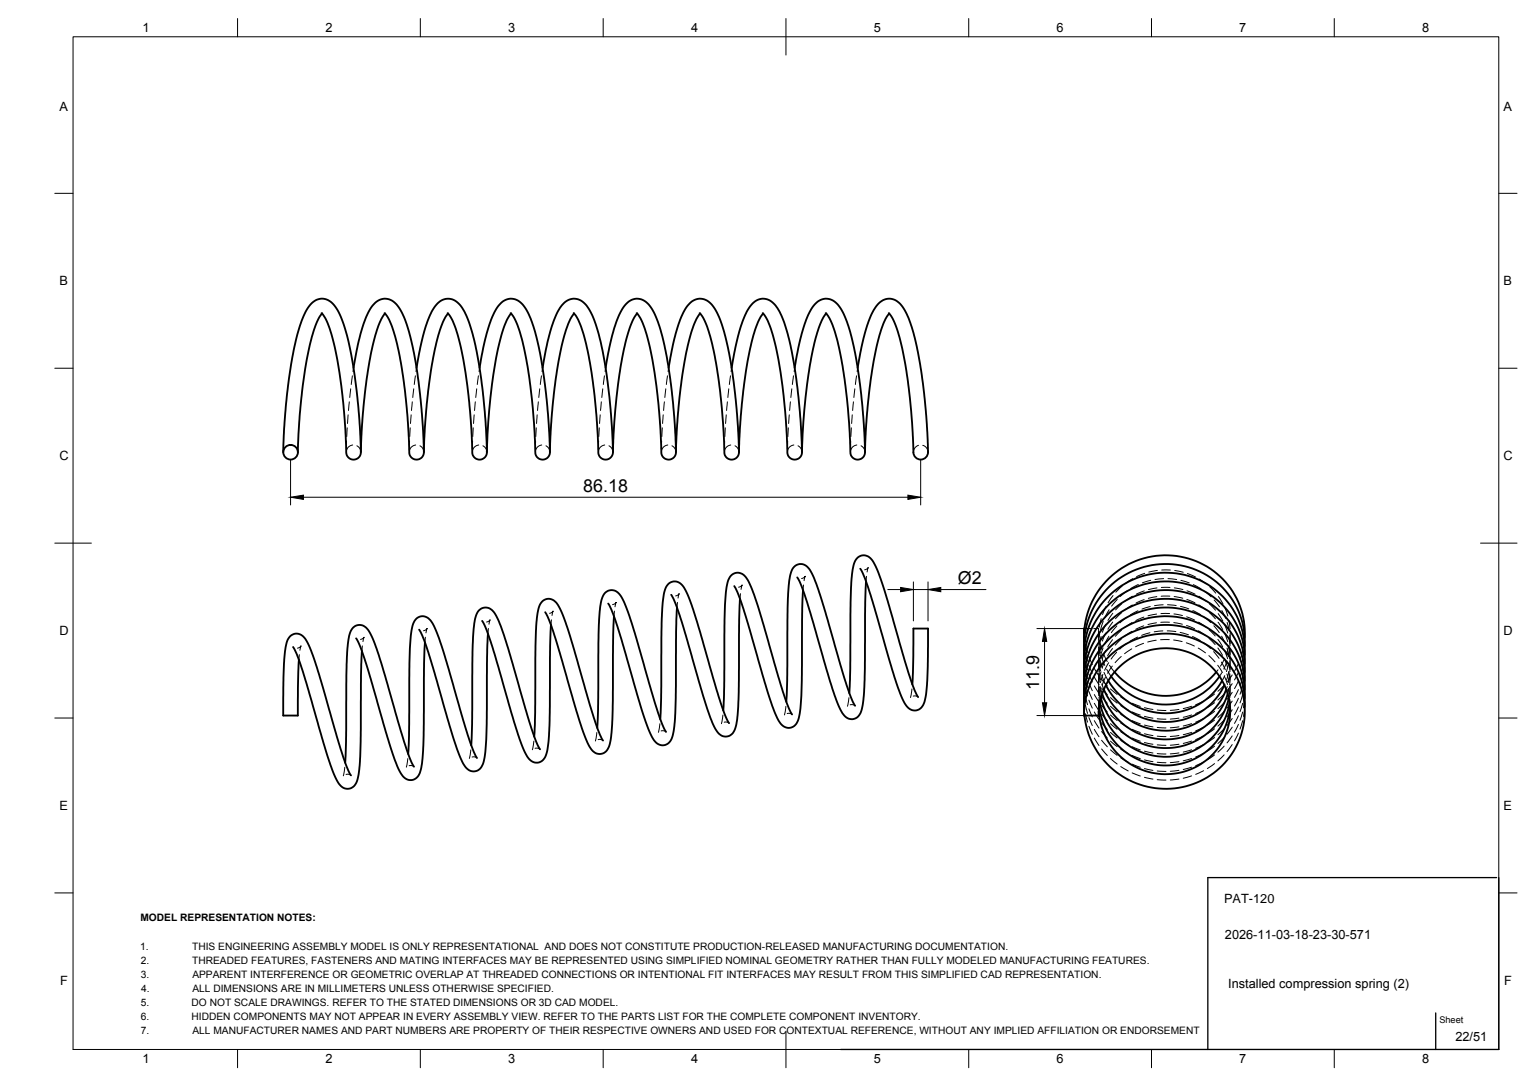
ISO-10303-21;
HEADER;
/* Generated by software containing ST-Developer
 * from STEP Tools, Inc. (www.steptools.com) 
 */

FILE_DESCRIPTION(
/* description */ ('Vibration shaker table dummy'),
/* implementation_level */ '2;1');

FILE_NAME(
/* name */ 'Installed compression spring (2).step',
/* time_stamp */ '2026-10-27T10:55:14-07:00',
/* author */ (''),
/* organization */ (''),
/* preprocessor_version */ 'ST-DEVELOPER v20.2',
/* originating_system */ 'Autodesk Translation Framework v15.17.0.0',
/* authorisation */ '');

FILE_SCHEMA (('AUTOMOTIVE_DESIGN { 1 0 10303 214 3 1 1 }'));
ENDSEC;

DATA;
#10=MECHANICAL_DESIGN_GEOMETRIC_PRESENTATION_REPRESENTATION('',(#703),#22394);
#588=B_SPLINE_CURVE_WITH_KNOTS('',3,(#19137,#19138,#19139,#19140,#19141,
#19142,#19143,#19144,#19145,#19146,#19147,#19148,#19149,#19150,#19151,#19152,
#19153,#19154,#19155,#19156,#19157,#19158,#19159,#19160,#19161,#19162,#19163,
#19164,#19165,#19166,#19167,#19168,#19169,#19170,#19171,#19172,#19173,#19174,
#19175,#19176,#19177,#19178,#19179,#19180,#19181,#19182,#19183,#19184,#19185,
#19186,#19187,#19188,#19189,#19190,#19191,#19192,#19193,#19194,#19195,#19196,
#19197,#19198,#19199,#19200,#19201,#19202,#19203,#19204,#19205,#19206,#19207,
#19208,#19209,#19210,#19211,#19212,#19213,#19214,#19215,#19216,#19217,#19218,
#19219,#19220,#19221,#19222,#19223,#19224,#19225,#19226,#19227,#19228,#19229,
#19230,#19231,#19232,#19233,#19234,#19235,#19236,#19237,#19238,#19239,#19240,
#19241,#19242,#19243,#19244,#19245,#19246,#19247,#19248,#19249,#19250,#19251,
#19252,#19253,#19254,#19255,#19256,#19257,#19258,#19259,#19260,#19261,#19262,
#19263,#19264,#19265,#19266,#19267,#19268,#19269,#19270,#19271,#19272,#19273,
#19274),.UNSPECIFIED.,.F.,.F.,(4,1,1,1,1,1,1,1,1,1,1,1,1,1,1,1,1,1,1,1,
1,1,1,1,1,1,1,1,1,1,1,1,1,1,1,1,1,1,1,1,1,1,1,1,1,1,1,1,1,1,1,1,1,1,1,1,
1,1,1,1,1,1,1,1,1,1,1,1,1,1,1,1,1,1,1,1,1,1,1,1,1,1,1,1,1,1,1,1,1,1,1,1,
1,1,1,1,1,1,1,1,1,1,1,1,1,1,1,1,1,1,1,1,1,1,1,1,1,1,1,1,1,1,1,1,1,1,1,1,
1,1,1,1,1,1,1,4),(0.,0.00892857142857143,0.0178571428571429,0.0267857142857143,
0.0357142857142857,0.0446428571428571,0.0535714285714286,0.0625,0.0714285714285714,
0.0803571428571428,0.0892857142857143,0.0982142857142857,0.107142857142857,
0.116071428571429,0.125,0.133928571428571,0.142857142857143,0.150793650793651,
0.154761904761905,0.156746031746032,0.158730158730159,0.166666666666667,
0.174603174603175,0.182539682539683,0.19047619047619,0.196428571428571,
0.202380952380952,0.208333333333333,0.214285714285714,0.222222222222222,
0.23015873015873,0.238095238095238,0.241071428571429,0.244047619047619,
0.25,0.255952380952381,0.261904761904762,0.267857142857143,0.273809523809524,
0.279761904761905,0.285714285714286,0.297619047619048,0.30952380952381,
0.321428571428571,0.327380952380952,0.333333333333333,0.341269841269841,
0.349206349206349,0.357142857142857,0.361111111111111,0.363095238095238,
0.365079365079365,0.373015873015873,0.380952380952381,0.386904761904762,
0.392857142857143,0.398809523809524,0.404761904761905,0.410714285714286,
0.416666666666667,0.422619047619048,0.428571428571429,0.4375,0.446428571428571,
0.455357142857143,0.459821428571429,0.464285714285714,0.470238095238095,
0.476190476190476,0.482142857142857,0.491071428571429,0.5,0.508928571428571,
0.517857142857143,0.526785714285714,0.535714285714286,0.544642857142857,
0.553571428571429,0.5625,0.571428571428571,0.580357142857143,0.589285714285714,
0.598214285714286,0.607142857142857,0.616071428571429,0.625,0.633928571428571,
0.642857142857143,0.650793650793651,0.658730158730159,0.666666666666667,
0.672619047619048,0.678571428571428,0.684523809523809,0.69047619047619,
0.696428571428571,0.702380952380952,0.708333333333333,0.714285714285714,
0.720238095238095,0.726190476190476,0.732142857142857,0.738095238095238,
0.744047619047619,0.75,0.755952380952381,0.761904761904762,0.76984126984127,
0.777777777777778,0.785714285714286,0.787946428571428,0.790178571428571,
0.794642857142857,0.803571428571428,0.8125,0.821428571428571,0.830357142857143,
0.839285714285714,0.848214285714286,0.857142857142857,0.866071428571429,
0.875,0.883928571428571,0.892857142857143,0.901785714285714,0.910714285714286,
0.919642857142857,0.928571428571429,0.9375,0.946428571428571,0.955357142857143,
0.964285714285714,0.973214285714286,0.982142857142857,0.991071428571429,
1.),.UNSPECIFIED.);
#592=B_SPLINE_SURFACE_WITH_KNOTS('',3,3,((#17754,#17755,#17756,#17757,#17758,
#17759,#17760,#17761,#17762,#17763,#17764,#17765,#17766,#17767,#17768,#17769,
#17770,#17771,#17772,#17773,#17774,#17775,#17776,#17777,#17778,#17779,#17780,
#17781,#17782,#17783,#17784,#17785,#17786,#17787,#17788,#17789,#17790,#17791,
#17792,#17793,#17794,#17795,#17796,#17797,#17798,#17799,#17800,#17801,#17802,
#17803,#17804,#17805,#17806,#17807,#17808,#17809,#17810,#17811,#17812,#17813,
#17814,#17815,#17816,#17817,#17818,#17819,#17820,#17821,#17822,#17823,#17824,
#17825,#17826,#17827,#17828,#17829,#17830,#17831,#17832,#17833,#17834,#17835,
#17836,#17837,#17838,#17839,#17840,#17841,#17842,#17843,#17844,#17845,#17846,
#17847,#17848,#17849,#17850,#17851,#17852,#17853,#17854,#17855,#17856,#17857,
#17858,#17859,#17860,#17861,#17862,#17863,#17864,#17865,#17866,#17867,#17868,
#17869,#17870,#17871,#17872,#17873,#17874,#17875,#17876,#17877,#17878,#17879,
#17880,#17881,#17882,#17883,#17884,#17885,#17886,#17887,#17888,#17889,#17890,
#17891),(#17892,#17893,#17894,#17895,#17896,#17897,#17898,#17899,#17900,
#17901,#17902,#17903,#17904,#17905,#17906,#17907,#17908,#17909,#17910,#17911,
#17912,#17913,#17914,#17915,#17916,#17917,#17918,#17919,#17920,#17921,#17922,
#17923,#17924,#17925,#17926,#17927,#17928,#17929,#17930,#17931,#17932,#17933,
#17934,#17935,#17936,#17937,#17938,#17939,#17940,#17941,#17942,#17943,#17944,
#17945,#17946,#17947,#17948,#17949,#17950,#17951,#17952,#17953,#17954,#17955,
#17956,#17957,#17958,#17959,#17960,#17961,#17962,#17963,#17964,#17965,#17966,
#17967,#17968,#17969,#17970,#17971,#17972,#17973,#17974,#17975,#17976,#17977,
#17978,#17979,#17980,#17981,#17982,#17983,#17984,#17985,#17986,#17987,#17988,
#17989,#17990,#17991,#17992,#17993,#17994,#17995,#17996,#17997,#17998,#17999,
#18000,#18001,#18002,#18003,#18004,#18005,#18006,#18007,#18008,#18009,#18010,
#18011,#18012,#18013,#18014,#18015,#18016,#18017,#18018,#18019,#18020,#18021,
#18022,#18023,#18024,#18025,#18026,#18027,#18028,#18029),(#18030,#18031,
#18032,#18033,#18034,#18035,#18036,#18037,#18038,#18039,#18040,#18041,#18042,
#18043,#18044,#18045,#18046,#18047,#18048,#18049,#18050,#18051,#18052,#18053,
#18054,#18055,#18056,#18057,#18058,#18059,#18060,#18061,#18062,#18063,#18064,
#18065,#18066,#18067,#18068,#18069,#18070,#18071,#18072,#18073,#18074,#18075,
#18076,#18077,#18078,#18079,#18080,#18081,#18082,#18083,#18084,#18085,#18086,
#18087,#18088,#18089,#18090,#18091,#18092,#18093,#18094,#18095,#18096,#18097,
#18098,#18099,#18100,#18101,#18102,#18103,#18104,#18105,#18106,#18107,#18108,
#18109,#18110,#18111,#18112,#18113,#18114,#18115,#18116,#18117,#18118,#18119,
#18120,#18121,#18122,#18123,#18124,#18125,#18126,#18127,#18128,#18129,#18130,
#18131,#18132,#18133,#18134,#18135,#18136,#18137,#18138,#18139,#18140,#18141,
#18142,#18143,#18144,#18145,#18146,#18147,#18148,#18149,#18150,#18151,#18152,
#18153,#18154,#18155,#18156,#18157,#18158,#18159,#18160,#18161,#18162,#18163,
#18164,#18165,#18166,#18167),(#18168,#18169,#18170,#18171,#18172,#18173,
#18174,#18175,#18176,#18177,#18178,#18179,#18180,#18181,#18182,#18183,#18184,
#18185,#18186,#18187,#18188,#18189,#18190,#18191,#18192,#18193,#18194,#18195,
#18196,#18197,#18198,#18199,#18200,#18201,#18202,#18203,#18204,#18205,#18206,
#18207,#18208,#18209,#18210,#18211,#18212,#18213,#18214,#18215,#18216,#18217,
#18218,#18219,#18220,#18221,#18222,#18223,#18224,#18225,#18226,#18227,#18228,
#18229,#18230,#18231,#18232,#18233,#18234,#18235,#18236,#18237,#18238,#18239,
#18240,#18241,#18242,#18243,#18244,#18245,#18246,#18247,#18248,#18249,#18250,
#18251,#18252,#18253,#18254,#18255,#18256,#18257,#18258,#18259,#18260,#18261,
#18262,#18263,#18264,#18265,#18266,#18267,#18268,#18269,#18270,#18271,#18272,
#18273,#18274,#18275,#18276,#18277,#18278,#18279,#18280,#18281,#18282,#18283,
#18284,#18285,#18286,#18287,#18288,#18289,#18290,#18291,#18292,#18293,#18294,
#18295,#18296,#18297,#18298,#18299,#18300,#18301,#18302,#18303,#18304,#18305),
(#18306,#18307,#18308,#18309,#18310,#18311,#18312,#18313,#18314,#18315,
#18316,#18317,#18318,#18319,#18320,#18321,#18322,#18323,#18324,#18325,#18326,
#18327,#18328,#18329,#18330,#18331,#18332,#18333,#18334,#18335,#18336,#18337,
#18338,#18339,#18340,#18341,#18342,#18343,#18344,#18345,#18346,#18347,#18348,
#18349,#18350,#18351,#18352,#18353,#18354,#18355,#18356,#18357,#18358,#18359,
#18360,#18361,#18362,#18363,#18364,#18365,#18366,#18367,#18368,#18369,#18370,
#18371,#18372,#18373,#18374,#18375,#18376,#18377,#18378,#18379,#18380,#18381,
#18382,#18383,#18384,#18385,#18386,#18387,#18388,#18389,#18390,#18391,#18392,
#18393,#18394,#18395,#18396,#18397,#18398,#18399,#18400,#18401,#18402,#18403,
#18404,#18405,#18406,#18407,#18408,#18409,#18410,#18411,#18412,#18413,#18414,
#18415,#18416,#18417,#18418,#18419,#18420,#18421,#18422,#18423,#18424,#18425,
#18426,#18427,#18428,#18429,#18430,#18431,#18432,#18433,#18434,#18435,#18436,
#18437,#18438,#18439,#18440,#18441,#18442,#18443),(#18444,#18445,#18446,
#18447,#18448,#18449,#18450,#18451,#18452,#18453,#18454,#18455,#18456,#18457,
#18458,#18459,#18460,#18461,#18462,#18463,#18464,#18465,#18466,#18467,#18468,
#18469,#18470,#18471,#18472,#18473,#18474,#18475,#18476,#18477,#18478,#18479,
#18480,#18481,#18482,#18483,#18484,#18485,#18486,#18487,#18488,#18489,#18490,
#18491,#18492,#18493,#18494,#18495,#18496,#18497,#18498,#18499,#18500,#18501,
#18502,#18503,#18504,#18505,#18506,#18507,#18508,#18509,#18510,#18511,#18512,
#18513,#18514,#18515,#18516,#18517,#18518,#18519,#18520,#18521,#18522,#18523,
#18524,#18525,#18526,#18527,#18528,#18529,#18530,#18531,#18532,#18533,#18534,
#18535,#18536,#18537,#18538,#18539,#18540,#18541,#18542,#18543,#18544,#18545,
#18546,#18547,#18548,#18549,#18550,#18551,#18552,#18553,#18554,#18555,#18556,
#18557,#18558,#18559,#18560,#18561,#18562,#18563,#18564,#18565,#18566,#18567,
#18568,#18569,#18570,#18571,#18572,#18573,#18574,#18575,#18576,#18577,#18578,
#18579,#18580,#18581),(#18582,#18583,#18584,#18585,#18586,#18587,#18588,
#18589,#18590,#18591,#18592,#18593,#18594,#18595,#18596,#18597,#18598,#18599,
#18600,#18601,#18602,#18603,#18604,#18605,#18606,#18607,#18608,#18609,#18610,
#18611,#18612,#18613,#18614,#18615,#18616,#18617,#18618,#18619,#18620,#18621,
#18622,#18623,#18624,#18625,#18626,#18627,#18628,#18629,#18630,#18631,#18632,
#18633,#18634,#18635,#18636,#18637,#18638,#18639,#18640,#18641,#18642,#18643,
#18644,#18645,#18646,#18647,#18648,#18649,#18650,#18651,#18652,#18653,#18654,
#18655,#18656,#18657,#18658,#18659,#18660,#18661,#18662,#18663,#18664,#18665,
#18666,#18667,#18668,#18669,#18670,#18671,#18672,#18673,#18674,#18675,#18676,
#18677,#18678,#18679,#18680,#18681,#18682,#18683,#18684,#18685,#18686,#18687,
#18688,#18689,#18690,#18691,#18692,#18693,#18694,#18695,#18696,#18697,#18698,
#18699,#18700,#18701,#18702,#18703,#18704,#18705,#18706,#18707,#18708,#18709,
#18710,#18711,#18712,#18713,#18714,#18715,#18716,#18717,#18718,#18719),
(#18720,#18721,#18722,#18723,#18724,#18725,#18726,#18727,#18728,#18729,
#18730,#18731,#18732,#18733,#18734,#18735,#18736,#18737,#18738,#18739,#18740,
#18741,#18742,#18743,#18744,#18745,#18746,#18747,#18748,#18749,#18750,#18751,
#18752,#18753,#18754,#18755,#18756,#18757,#18758,#18759,#18760,#18761,#18762,
#18763,#18764,#18765,#18766,#18767,#18768,#18769,#18770,#18771,#18772,#18773,
#18774,#18775,#18776,#18777,#18778,#18779,#18780,#18781,#18782,#18783,#18784,
#18785,#18786,#18787,#18788,#18789,#18790,#18791,#18792,#18793,#18794,#18795,
#18796,#18797,#18798,#18799,#18800,#18801,#18802,#18803,#18804,#18805,#18806,
#18807,#18808,#18809,#18810,#18811,#18812,#18813,#18814,#18815,#18816,#18817,
#18818,#18819,#18820,#18821,#18822,#18823,#18824,#18825,#18826,#18827,#18828,
#18829,#18830,#18831,#18832,#18833,#18834,#18835,#18836,#18837,#18838,#18839,
#18840,#18841,#18842,#18843,#18844,#18845,#18846,#18847,#18848,#18849,#18850,
#18851,#18852,#18853,#18854,#18855,#18856,#18857),(#18858,#18859,#18860,
#18861,#18862,#18863,#18864,#18865,#18866,#18867,#18868,#18869,#18870,#18871,
#18872,#18873,#18874,#18875,#18876,#18877,#18878,#18879,#18880,#18881,#18882,
#18883,#18884,#18885,#18886,#18887,#18888,#18889,#18890,#18891,#18892,#18893,
#18894,#18895,#18896,#18897,#18898,#18899,#18900,#18901,#18902,#18903,#18904,
#18905,#18906,#18907,#18908,#18909,#18910,#18911,#18912,#18913,#18914,#18915,
#18916,#18917,#18918,#18919,#18920,#18921,#18922,#18923,#18924,#18925,#18926,
#18927,#18928,#18929,#18930,#18931,#18932,#18933,#18934,#18935,#18936,#18937,
#18938,#18939,#18940,#18941,#18942,#18943,#18944,#18945,#18946,#18947,#18948,
#18949,#18950,#18951,#18952,#18953,#18954,#18955,#18956,#18957,#18958,#18959,
#18960,#18961,#18962,#18963,#18964,#18965,#18966,#18967,#18968,#18969,#18970,
#18971,#18972,#18973,#18974,#18975,#18976,#18977,#18978,#18979,#18980,#18981,
#18982,#18983,#18984,#18985,#18986,#18987,#18988,#18989,#18990,#18991,#18992,
#18993,#18994,#18995),(#18996,#18997,#18998,#18999,#19000,#19001,#19002,
#19003,#19004,#19005,#19006,#19007,#19008,#19009,#19010,#19011,#19012,#19013,
#19014,#19015,#19016,#19017,#19018,#19019,#19020,#19021,#19022,#19023,#19024,
#19025,#19026,#19027,#19028,#19029,#19030,#19031,#19032,#19033,#19034,#19035,
#19036,#19037,#19038,#19039,#19040,#19041,#19042,#19043,#19044,#19045,#19046,
#19047,#19048,#19049,#19050,#19051,#19052,#19053,#19054,#19055,#19056,#19057,
#19058,#19059,#19060,#19061,#19062,#19063,#19064,#19065,#19066,#19067,#19068,
#19069,#19070,#19071,#19072,#19073,#19074,#19075,#19076,#19077,#19078,#19079,
#19080,#19081,#19082,#19083,#19084,#19085,#19086,#19087,#19088,#19089,#19090,
#19091,#19092,#19093,#19094,#19095,#19096,#19097,#19098,#19099,#19100,#19101,
#19102,#19103,#19104,#19105,#19106,#19107,#19108,#19109,#19110,#19111,#19112,
#19113,#19114,#19115,#19116,#19117,#19118,#19119,#19120,#19121,#19122,#19123,
#19124,#19125,#19126,#19127,#19128,#19129,#19130,#19131,#19132,#19133)),
 .UNSPECIFIED.,.T.,.F.,.F.,(4,1,1,1,1,1,1,4),(4,1,1,1,1,1,1,1,1,1,1,1,1,
1,1,1,1,1,1,1,1,1,1,1,1,1,1,1,1,1,1,1,1,1,1,1,1,1,1,1,1,1,1,1,1,1,1,1,1,
1,1,1,1,1,1,1,1,1,1,1,1,1,1,1,1,1,1,1,1,1,1,1,1,1,1,1,1,1,1,1,1,1,1,1,1,
1,1,1,1,1,1,1,1,1,1,1,1,1,1,1,1,1,1,1,1,1,1,1,1,1,1,1,1,1,1,1,1,1,1,1,1,
1,1,1,1,1,1,1,1,1,1,1,1,1,1,4),(-3.14159265358979,-2.24399475256414,-1.34639685153848,
-0.448798950512828,0.448798950512828,1.34639685153848,2.24399475256414,
3.14159265358979),(0.,0.00892857142857143,0.0178571428571429,0.0267857142857143,
0.0357142857142857,0.0446428571428571,0.0535714285714286,0.0625,0.0714285714285714,
0.0803571428571428,0.0892857142857143,0.0982142857142857,0.107142857142857,
0.116071428571429,0.125,0.133928571428571,0.142857142857143,0.150793650793651,
0.154761904761905,0.156746031746032,0.158730158730159,0.166666666666667,
0.174603174603175,0.182539682539683,0.19047619047619,0.196428571428571,
0.202380952380952,0.208333333333333,0.214285714285714,0.222222222222222,
0.23015873015873,0.238095238095238,0.241071428571429,0.244047619047619,
0.25,0.255952380952381,0.261904761904762,0.267857142857143,0.273809523809524,
0.279761904761905,0.285714285714286,0.297619047619048,0.30952380952381,
0.321428571428571,0.327380952380952,0.333333333333333,0.341269841269841,
0.349206349206349,0.357142857142857,0.361111111111111,0.363095238095238,
0.365079365079365,0.373015873015873,0.380952380952381,0.386904761904762,
0.392857142857143,0.398809523809524,0.404761904761905,0.410714285714286,
0.416666666666667,0.422619047619048,0.428571428571429,0.4375,0.446428571428571,
0.455357142857143,0.459821428571429,0.464285714285714,0.470238095238095,
0.476190476190476,0.482142857142857,0.491071428571429,0.5,0.508928571428571,
0.517857142857143,0.526785714285714,0.535714285714286,0.544642857142857,
0.553571428571429,0.5625,0.571428571428571,0.580357142857143,0.589285714285714,
0.598214285714286,0.607142857142857,0.616071428571429,0.625,0.633928571428571,
0.642857142857143,0.650793650793651,0.658730158730159,0.666666666666667,
0.672619047619048,0.678571428571428,0.684523809523809,0.69047619047619,
0.696428571428571,0.702380952380952,0.708333333333333,0.714285714285714,
0.720238095238095,0.726190476190476,0.732142857142857,0.738095238095238,
0.744047619047619,0.75,0.755952380952381,0.761904761904762,0.76984126984127,
0.777777777777778,0.785714285714286,0.787946428571428,0.790178571428571,
0.794642857142857,0.803571428571428,0.8125,0.821428571428571,0.830357142857143,
0.839285714285714,0.848214285714286,0.857142857142857,0.866071428571429,
0.875,0.883928571428571,0.892857142857143,0.901785714285714,0.910714285714286,
0.919642857142857,0.928571428571429,0.9375,0.946428571428571,0.955357142857143,
0.964285714285714,0.973214285714286,0.982142857142857,0.991071428571429,
1.),.UNSPECIFIED.);
#611=SHAPE_REPRESENTATION_RELATIONSHIP('SRR','None',#22657,#657);
#657=ADVANCED_BREP_SHAPE_REPRESENTATION('',(#749),#22363);
#703=STYLED_ITEM('',(#22961),#749);
#749=MANIFOLD_SOLID_BREP('Body1',#9221);
#1168=PLANE('',#10140);
#1169=PLANE('',#10141);
#1529=FACE_OUTER_BOUND('',#2157,.T.);
#1530=FACE_OUTER_BOUND('',#2158,.T.);
#1531=FACE_OUTER_BOUND('',#2159,.T.);
#2157=EDGE_LOOP('',(#7122,#7123,#7124,#7125));
#2158=EDGE_LOOP('',(#7126));
#2159=EDGE_LOOP('',(#7127));
#4032=CIRCLE('',#10138,0.1);
#4033=CIRCLE('',#10139,0.1);
#4659=VERTEX_POINT('',#19134);
#4660=VERTEX_POINT('',#19136);
#5554=EDGE_CURVE('',#4659,#4659,#4032,.T.);
#5555=EDGE_CURVE('',#4659,#4660,#588,.T.);
#5556=EDGE_CURVE('',#4660,#4660,#4033,.T.);
#7122=ORIENTED_EDGE('',*,*,#5554,.T.);
#7123=ORIENTED_EDGE('',*,*,#5555,.T.);
#7124=ORIENTED_EDGE('',*,*,#5556,.F.);
#7125=ORIENTED_EDGE('',*,*,#5555,.F.);
#7126=ORIENTED_EDGE('',*,*,#5556,.T.);
#7127=ORIENTED_EDGE('',*,*,#5554,.F.);
#8894=ADVANCED_FACE('',(#1529),#592,.T.);
#8895=ADVANCED_FACE('',(#1530),#1168,.T.);
#8896=ADVANCED_FACE('',(#1531),#1169,.F.);
#9221=CLOSED_SHELL('',(#8894,#8895,#8896));
#10137=AXIS2_PLACEMENT_3D('',#17753,#11968,#11969);
#10138=AXIS2_PLACEMENT_3D('',#19135,#11970,#11971);
#10139=AXIS2_PLACEMENT_3D('',#19275,#11972,#11973);
#10140=AXIS2_PLACEMENT_3D('',#19276,#11974,#11975);
#10141=AXIS2_PLACEMENT_3D('',#19277,#11976,#11977);
#11968=DIRECTION('axis',(0.,0.,1.));
#11969=DIRECTION('refdir',(1.,0.,0.));
#11970=DIRECTION('center_axis',(-0.000133356257939316,0.990604928518337,
0.136754735973894));
#11971=DIRECTION('ref_axis',(1.84100635426204E-5,-0.136754734734703,0.990604937494615));
#11972=DIRECTION('center_axis',(0.000133356514931307,0.990604928490669,
0.136754736174063));
#11973=DIRECTION('ref_axis',(-0.722226697922822,0.0946826992832939,-0.68514508190888));
#11974=DIRECTION('center_axis',(0.000133356514931307,0.990604928490669,
0.136754736174063));
#11975=DIRECTION('ref_axis',(-0.722226697922822,0.0946826992832939,-0.68514508190888));
#11976=DIRECTION('center_axis',(-0.000133356257939316,0.990604928518337,
0.136754735973894));
#11977=DIRECTION('ref_axis',(1.84100635426204E-5,-0.136754734734703,0.990604937494615));
#17753=CARTESIAN_POINT('',(0.,0.,0.));
#17754=CARTESIAN_POINT('Ctrl Pts',(6.99999815899365,-3.98632452652653,2.60093950625054));
#17755=CARTESIAN_POINT('Ctrl Pts',(6.99997288064459,-3.79855038269031,2.62686205390176));
#17756=CARTESIAN_POINT('Ctrl Pts',(6.89233514047511,-3.42414397295474,2.67881370715146));
#17757=CARTESIAN_POINT('Ctrl Pts',(6.45271448161715,-3.02998089899105,2.757384351524));
#17758=CARTESIAN_POINT('Ctrl Pts',(5.86671979479608,-2.93006055988124,2.83651312593273));
#17759=CARTESIAN_POINT('Ctrl Pts',(5.31329781017118,-3.15858496371257,2.91622300969429));
#17760=CARTESIAN_POINT('Ctrl Pts',(4.9638387202763,-3.65012742948249,2.99648818069946));
#17761=CARTESIAN_POINT('Ctrl Pts',(4.9293710419426,-4.25616717719541,3.07729927110974));
#17762=CARTESIAN_POINT('Ctrl Pts',(5.22419213535424,-4.79140012919127,3.15863486906283));
#17763=CARTESIAN_POINT('Ctrl Pts',(5.76222069265107,-5.08919945404236,3.24047453667969));
#17764=CARTESIAN_POINT('Ctrl Pts',(6.379677030618,-5.05504702300603,3.32279319426342));
#17765=CARTESIAN_POINT('Ctrl Pts',(6.88712884688249,-4.6955749219134,3.40556355651458));
#17766=CARTESIAN_POINT('Ctrl Pts',(7.12670085302573,-4.11831918936923,3.48875539197247));
#17767=CARTESIAN_POINT('Ctrl Pts',(7.02192637673817,-3.49920475943206,3.57233609217612));
#17768=CARTESIAN_POINT('Ctrl Pts',(6.60200480535371,-3.02877356919622,3.65627071403784));
#17769=CARTESIAN_POINT('Ctrl Pts',(5.99389696970595,-2.85326346917548,3.74052223770667));
#17770=CARTESIAN_POINT('Ctrl Pts',(5.38356210524816,-3.02876561374954,3.82505176545516));
#17771=CARTESIAN_POINT('Ctrl Pts',(4.97486808401256,-3.48597581907603,3.90667922332894));
#17772=CARTESIAN_POINT('Ctrl Pts',(4.87764331063032,-3.96854834063101,3.97275270796177));
#17773=CARTESIAN_POINT('Ctrl Pts',(4.93363491104256,-4.28466096216571,4.01685604464165));
#17774=CARTESIAN_POINT('Ctrl Pts',(4.99817931143911,-4.45530970670709,4.04207155735716));
#17775=CARTESIAN_POINT('Ctrl Pts',(5.12597275373369,-4.69744865131441,4.07990746653167));
#17776=CARTESIAN_POINT('Ctrl Pts',(5.42875069944469,-4.99309340796393,4.13670511444809));
#17777=CARTESIAN_POINT('Ctrl Pts',(5.97231920216535,-5.14605898976926,4.21249748606625));
#17778=CARTESIAN_POINT('Ctrl Pts',(6.52320508223107,-5.02044374257342,4.28832048254892));
#17779=CARTESIAN_POINT('Ctrl Pts',(6.91110467076896,-4.67743260856581,4.35782392841035));
#17780=CARTESIAN_POINT('Ctrl Pts',(7.09644745188598,-4.25185787791867,4.42098501720712));
#17781=CARTESIAN_POINT('Ctrl Pts',(7.11227598252982,-3.83457932502243,4.47779828333078));
#17782=CARTESIAN_POINT('Ctrl Pts',(6.97422198867159,-3.44096105119827,4.53456659991209));
#17783=CARTESIAN_POINT('Ctrl Pts',(6.67241777459347,-3.08955752755044,4.59757801617794));
#17784=CARTESIAN_POINT('Ctrl Pts',(6.20242890124212,-2.8776477149725,4.66678930738527));
#17785=CARTESIAN_POINT('Ctrl Pts',(5.64251878205079,-2.91980762281901,4.74213608937642));
#17786=CARTESIAN_POINT('Ctrl Pts',(5.2704159386044,-3.1605530148329,4.80163845364204));
#17787=CARTESIAN_POINT('Ctrl Pts',(5.0774166278585,-3.41255654376288,4.84539629257686));
#17788=CARTESIAN_POINT('Ctrl Pts',(4.95479769651029,-3.65506677262475,4.88286085266752));
#17789=CARTESIAN_POINT('Ctrl Pts',(4.89096164216428,-3.99267527518354,4.9296088561907));
#17790=CARTESIAN_POINT('Ctrl Pts',(4.9676452372308,-4.39667000889553,4.98556279567646));
#17791=CARTESIAN_POINT('Ctrl Pts',(5.18583996189851,-4.74396038265063,5.04136211338706));
#17792=CARTESIAN_POINT('Ctrl Pts',(5.51489715544512,-4.98648283834255,5.09699623582978));
#17793=CARTESIAN_POINT('Ctrl Pts',(5.90877797642046,-5.0921366099034,5.15245506500268));
#17794=CARTESIAN_POINT('Ctrl Pts',(6.31208382647452,-5.04618505638536,5.20772889790527));
#17795=CARTESIAN_POINT('Ctrl Pts',(6.79039563711824,-4.79482787477752,5.28116853494519));
#17796=CARTESIAN_POINT('Ctrl Pts',(7.14364250607538,-4.18339760328549,5.37246079320281));
#17797=CARTESIAN_POINT('Ctrl Pts',(6.95465392442801,-3.3615290602033,5.48113680479085));
#17798=CARTESIAN_POINT('Ctrl Pts',(6.37954281770185,-2.97211167108618,5.57092649504958));
#17799=CARTESIAN_POINT('Ctrl Pts',(5.85508217241069,-2.95446460563552,5.64227218334414));
#17800=CARTESIAN_POINT('Ctrl Pts',(5.44460306454923,-3.0974244576334,5.70145206942602));
#17801=CARTESIAN_POINT('Ctrl Pts',(5.09938139322235,-3.43453521092238,5.76619150122483));
#17802=CARTESIAN_POINT('Ctrl Pts',(4.94592320318296,-3.93442474869926,5.83636208316637));
#17803=CARTESIAN_POINT('Ctrl Pts',(5.03197265676116,-4.35840627465708,5.89445465107149));
#17804=CARTESIAN_POINT('Ctrl Pts',(5.19219264369348,-4.60564299044654,5.93491706685731));
#17805=CARTESIAN_POINT('Ctrl Pts',(5.30719577297855,-4.72651611720447,5.95798055540973));
#17806=CARTESIAN_POINT('Ctrl Pts',(5.50053046023923,-4.88495348501329,5.99251787759586));
#17807=CARTESIAN_POINT('Ctrl Pts',(5.85832951556707,-5.02507253962729,6.04410658286047));
#17808=CARTESIAN_POINT('Ctrl Pts',(6.32126493019694,-4.96668267597821,6.10673564915363));
#17809=CARTESIAN_POINT('Ctrl Pts',(6.67328517320073,-4.74489735077078,6.1633365491453));
#17810=CARTESIAN_POINT('Ctrl Pts',(6.89435900913716,-4.44516759248262,6.21402149084589));
#17811=CARTESIAN_POINT('Ctrl Pts',(6.99016055458223,-4.08705298460299,6.26445344730346));
#17812=CARTESIAN_POINT('Ctrl Pts',(6.94870527391535,-3.72056310115263,6.31463598339954));
#17813=CARTESIAN_POINT('Ctrl Pts',(6.77696548585144,-3.39623351183634,6.36457330966794));
#17814=CARTESIAN_POINT('Ctrl Pts',(6.50006848678236,-3.15797695360399,6.41427030439494));
#17815=CARTESIAN_POINT('Ctrl Pts',(6.15689079921747,-3.03828948600061,6.46373243937456));
#17816=CARTESIAN_POINT('Ctrl Pts',(5.73494713487383,-3.05387392617641,6.52117143017342));
#17817=CARTESIAN_POINT('Ctrl Pts',(5.30575107583077,-3.29070893773119,6.58644590514151));
#17818=CARTESIAN_POINT('Ctrl Pts',(5.04125313845857,-3.77122732190886,6.6594050878354));
#17819=CARTESIAN_POINT('Ctrl Pts',(5.06714113786846,-4.2240700226978,6.71983222627245));
#17820=CARTESIAN_POINT('Ctrl Pts',(5.22896371026909,-4.53583531846688,6.76796591127916));
#17821=CARTESIAN_POINT('Ctrl Pts',(5.42916113979845,-4.74785467675554,6.80796630808184));
#17822=CARTESIAN_POINT('Ctrl Pts',(5.714367370309,-4.89850759732021,6.85183024025803));
#17823=CARTESIAN_POINT('Ctrl Pts',(6.06253639457921,-4.93755475445945,6.89952195690528));
#17824=CARTESIAN_POINT('Ctrl Pts',(6.4565847787629,-4.83233977440753,6.95498839066731));
#17825=CARTESIAN_POINT('Ctrl Pts',(6.81022730237302,-4.51633849133825,7.01814871600544));
#17826=CARTESIAN_POINT('Ctrl Pts',(6.95706828830077,-4.00489886911992,7.08893287981098));
#17827=CARTESIAN_POINT('Ctrl Pts',(6.81021224891959,-3.49584469103884,7.15948666255227));
#17828=CARTESIAN_POINT('Ctrl Pts',(6.41592301667082,-3.14352189275395,7.22985222727915));
#17829=CARTESIAN_POINT('Ctrl Pts',(5.89582428767248,-3.0555832223308,7.30007283378182));
#17830=CARTESIAN_POINT('Ctrl Pts',(5.40914881608276,-3.25711226719962,7.37019262219717));
#17831=CARTESIAN_POINT('Ctrl Pts',(5.10471600640629,-3.68647088534127,7.4402563254545));
#17832=CARTESIAN_POINT('Ctrl Pts',(5.07493689936822,-4.21187381141773,7.51030900528994));
#17833=CARTESIAN_POINT('Ctrl Pts',(5.32972438815395,-4.67276168571651,7.58039577687912));
#17834=CARTESIAN_POINT('Ctrl Pts',(5.79102554371443,-4.92784792737786,7.65056157421906));
#17835=CARTESIAN_POINT('Ctrl Pts',(6.31826031255578,-4.89837953861158,7.72085085714204));
#17836=CARTESIAN_POINT('Ctrl Pts',(6.75020660471299,-4.59231290695902,7.79130734550421));
#17837=CARTESIAN_POINT('Ctrl Pts',(6.95334524231267,-4.10180979072915,7.86197377515194));
#17838=CARTESIAN_POINT('Ctrl Pts',(6.86452811856373,-3.57660445666216,7.93289164673106));
#17839=CARTESIAN_POINT('Ctrl Pts',(6.50822949801913,-3.17741851765368,8.00410096472273));
#17840=CARTESIAN_POINT('Ctrl Pts',(5.99202912111436,-3.02846879700038,8.07564001126929));
#17841=CARTESIAN_POINT('Ctrl Pts',(5.47262775862424,-3.1772786287127,8.14754510192845));
#17842=CARTESIAN_POINT('Ctrl Pts',(5.12396773984527,-3.56713104102442,8.21717245978697));
#17843=CARTESIAN_POINT('Ctrl Pts',(5.02465088008016,-4.0589090579052,8.28449962671212));
#17844=CARTESIAN_POINT('Ctrl Pts',(5.16664179671633,-4.52183049710153,8.34949563002517));
#17845=CARTESIAN_POINT('Ctrl Pts',(5.48622133819085,-4.83366725020512,8.40942447534479));
#17846=CARTESIAN_POINT('Ctrl Pts',(5.86625745021743,-4.9665851067969,8.4641954747342));
#17847=CARTESIAN_POINT('Ctrl Pts',(6.22997586892847,-4.95324406413884,8.5137197914407));
#17848=CARTESIAN_POINT('Ctrl Pts',(6.56523678307791,-4.80705258085916,8.56348049146453));
#17849=CARTESIAN_POINT('Ctrl Pts',(6.8252178463785,-4.54733568382595,8.61348288991823));
#17850=CARTESIAN_POINT('Ctrl Pts',(6.97306928054101,-4.20890471076454,8.6637316832973));
#17851=CARTESIAN_POINT('Ctrl Pts',(6.98712341108126,-3.83802816814003,8.7142309149468));
#17852=CARTESIAN_POINT('Ctrl Pts',(6.86409431800442,-3.4858887373625,8.76498396878373));
#17853=CARTESIAN_POINT('Ctrl Pts',(6.61968641501593,-3.20161333099039,8.81599356080702));
#17854=CARTESIAN_POINT('Ctrl Pts',(6.28663539552411,-3.02539046352671,8.8672617337013));
#17855=CARTESIAN_POINT('Ctrl Pts',(5.91032079687008,-2.98281618785264,8.9187898484193));
#17856=CARTESIAN_POINT('Ctrl Pts',(5.54261902100133,-3.08115683102349,8.97057858319571));
#17857=CARTESIAN_POINT('Ctrl Pts',(5.23470149593991,-3.30818973404657,9.02262792887906));
#17858=CARTESIAN_POINT('Ctrl Pts',(5.03002953653242,-3.63360637314209,9.07493719454492));
#17859=CARTESIAN_POINT('Ctrl Pts',(4.95795339049146,-4.01324887545392,9.12750499722226));
#17860=CARTESIAN_POINT('Ctrl Pts',(5.03008733681497,-4.39465616925505,9.18032929191999));
#17861=CARTESIAN_POINT('Ctrl Pts',(5.26037098227884,-4.76198737973904,9.23930488376548));
#17862=CARTESIAN_POINT('Ctrl Pts',(5.66815402132354,-5.02611715334513,9.30453505328307));
#17863=CARTESIAN_POINT('Ctrl Pts',(6.20031175950905,-5.06610553161693,9.37613052247429));
#17864=CARTESIAN_POINT('Ctrl Pts',(6.57211483447548,-4.89867154701958,9.43089482659667));
#17865=CARTESIAN_POINT('Ctrl Pts',(6.77268428325753,-4.71398594666241,9.46854124254023));
#17866=CARTESIAN_POINT('Ctrl Pts',(6.89732261541234,-4.56210906285714,9.4956893772699));
#17867=CARTESIAN_POINT('Ctrl Pts',(7.05743952416135,-4.25373892219051,9.54330952558428));
#17868=CARTESIAN_POINT('Ctrl Pts',(7.08681427060224,-3.7413976498585,9.61164803498953));
#17869=CARTESIAN_POINT('Ctrl Pts',(6.78743967682059,-3.19877575055479,9.69412425474241));
#17870=CARTESIAN_POINT('Ctrl Pts',(6.24245837315985,-2.89706443193603,9.77704206668623));
#17871=CARTESIAN_POINT('Ctrl Pts',(5.61746900273164,-2.93185417099466,9.86037047868398));
#17872=CARTESIAN_POINT('Ctrl Pts',(5.1042042416184,-3.29518411512121,9.94407604361117));
#17873=CARTESIAN_POINT('Ctrl Pts',(4.86233946758306,-3.8785536270643,10.0281231251224));
#17874=CARTESIAN_POINT('Ctrl Pts',(4.96816269898698,-4.50332086698013,10.1124740074888));
#17875=CARTESIAN_POINT('Ctrl Pts',(5.3915816199262,-4.97752738430232,10.1970892227568));
#17876=CARTESIAN_POINT('Ctrl Pts',(6.00397807691952,-5.15417755509278,10.281927720062));
#17877=CARTESIAN_POINT('Ctrl Pts',(6.61779621608409,-4.97752665860305,10.3669471357688));
#17878=CARTESIAN_POINT('Ctrl Pts',(7.04418758947222,-4.50057596349951,10.4521040140405));
#17879=CARTESIAN_POINT('Ctrl Pts',(7.15154318711507,-3.86917823804319,10.5373541207604));
#17880=CARTESIAN_POINT('Ctrl Pts',(6.9063217242137,-3.27712490715728,10.622652644332));
#17881=CARTESIAN_POINT('Ctrl Pts',(6.38365961018741,-2.90630232377856,10.70795449752));
#17882=CARTESIAN_POINT('Ctrl Pts',(5.74407957751689,-2.87046702674317,10.7932145497474));
#17883=CARTESIAN_POINT('Ctrl Pts',(5.18413779010185,-3.18009512220889,10.8783879953558));
#17884=CARTESIAN_POINT('Ctrl Pts',(4.87504525063398,-3.73939474085648,10.9634303821887));
#17885=CARTESIAN_POINT('Ctrl Pts',(4.9113280193628,-4.37593360867611,11.0482983399598));
#17886=CARTESIAN_POINT('Ctrl Pts',(5.27937248430205,-4.89450749674953,11.1329488708158));
#17887=CARTESIAN_POINT('Ctrl Pts',(5.86527624347711,-5.13679808752952,11.2173417295453));
#17888=CARTESIAN_POINT('Ctrl Pts',(6.48799534199112,-5.03087191620999,11.3014349903219));
#17889=CARTESIAN_POINT('Ctrl Pts',(6.95693136473707,-4.61090781293032,11.3851957485584));
#17890=CARTESIAN_POINT('Ctrl Pts',(7.07219562678886,-4.21035033769926,11.4407823887657));
#17891=CARTESIAN_POINT('Ctrl Pts',(7.07222266979228,-4.00946826992833,11.4685145081909));
#17892=CARTESIAN_POINT('Ctrl Pts',(6.97007822923057,-3.98632855437836,2.60093950625054));
#17893=CARTESIAN_POINT('Ctrl Pts',(6.97005368434428,-3.80400276250044,2.62610989942311));
#17894=CARTESIAN_POINT('Ctrl Pts',(6.8655981616237,-3.44058276592777,2.67653039560817));
#17895=CARTESIAN_POINT('Ctrl Pts',(6.43867935390673,-3.05771294402619,2.75283688635242));
#17896=CARTESIAN_POINT('Ctrl Pts',(5.86925370182103,-2.96056862970221,2.829722772863));
#17897=CARTESIAN_POINT('Ctrl Pts',(5.33104067083453,-3.18273229632189,2.90723423398096));
#17898=CARTESIAN_POINT('Ctrl Pts',(4.99083036824212,-3.6611258102588,2.98535322301203));
#17899=CARTESIAN_POINT('Ctrl Pts',(4.95715560557959,-4.25162171008957,3.06408756320453));
#17900=CARTESIAN_POINT('Ctrl Pts',(5.24465534103322,-4.77378946224153,3.14342202919564));
#17901=CARTESIAN_POINT('Ctrl Pts',(5.77010719210167,-5.06476100581107,3.22334344667496));
#17902=CARTESIAN_POINT('Ctrl Pts',(6.37406294588003,-5.0314844936736,3.30385018064892));
#17903=CARTESIAN_POINT('Ctrl Pts',(6.87124480480666,-4.67945377128695,3.38491957776513));
#17904=CARTESIAN_POINT('Ctrl Pts',(7.10644641749634,-4.11311294816235,3.46653370137737));
#17905=CARTESIAN_POINT('Ctrl Pts',(7.00362219975504,-3.50458520131084,3.54866794881851));
#17906=CARTESIAN_POINT('Ctrl Pts',(6.59028971235191,-3.04128632982343,3.63129605781087));
#17907=CARTESIAN_POINT('Ctrl Pts',(5.9904902635316,-2.86799412215644,3.71438857179753));
#17908=CARTESIAN_POINT('Ctrl Pts',(5.38725457312936,-3.04126659406085,3.79791248632923));
#17909=CARTESIAN_POINT('Ctrl Pts',(4.98243162058577,-3.49388688470476,3.87872607649656));
#17910=CARTESIAN_POINT('Ctrl Pts',(4.88586987972222,-3.97261107956554,3.94426166404564));
#17911=CARTESIAN_POINT('Ctrl Pts',(4.94147690622331,-4.28666010423245,3.9880717841222));
#17912=CARTESIAN_POINT('Ctrl Pts',(5.00564118171601,-4.45631175436491,4.01313856907925));
#17913=CARTESIAN_POINT('Ctrl Pts',(5.13273792342617,-4.69714409310281,4.05076810237111));
#17914=CARTESIAN_POINT('Ctrl Pts',(5.43409624307086,-4.99155886825263,4.10729667550138));
#17915=CARTESIAN_POINT('Ctrl Pts',(5.97628316486736,-5.1442798788599,4.18289693437406));
#17916=CARTESIAN_POINT('Ctrl Pts',(6.52681800343661,-5.01887678936212,4.25865819770454));
#17917=CARTESIAN_POINT('Ctrl Pts',(6.91522840587363,-4.67558077820218,4.32822383176324));
#17918=CARTESIAN_POINT('Ctrl Pts',(7.10113200959162,-4.24885108696776,4.39155418341742));
#17919=CARTESIAN_POINT('Ctrl Pts',(7.11708265563879,-3.82987437918727,4.44859070552638));
#17920=CARTESIAN_POINT('Ctrl Pts',(6.97831413390946,-3.43409394973361,4.50566173126832));
#17921=CARTESIAN_POINT('Ctrl Pts',(6.6745131582099,-3.08027116188779,4.56909239590932));
#17922=CARTESIAN_POINT('Ctrl Pts',(6.2006354612538,-2.86648985101506,4.63887572589507));
#17923=CARTESIAN_POINT('Ctrl Pts',(5.63505204541033,-2.90895569779608,4.71498055830681));
#17924=CARTESIAN_POINT('Ctrl Pts',(5.25855479608114,-3.15244878707084,4.77515896552872));
#17925=CARTESIAN_POINT('Ctrl Pts',(5.06304540191057,-3.4077178457721,4.81948131645844));
#17926=CARTESIAN_POINT('Ctrl Pts',(4.93875890697152,-3.65351683513821,4.85745130169426));
#17927=CARTESIAN_POINT('Ctrl Pts',(4.87395928312855,-3.99601029957039,4.9048726153362));
#17928=CARTESIAN_POINT('Ctrl Pts',(4.95180908604431,-4.40634593719688,4.961698237853));
#17929=CARTESIAN_POINT('Ctrl Pts',(5.17363722686749,-4.75950452494967,5.01843134223497));
#17930=CARTESIAN_POINT('Ctrl Pts',(5.50858725429261,-5.00640760956707,5.07505875580519));
#17931=CARTESIAN_POINT('Ctrl Pts',(5.90996241751456,-5.11411410956675,5.13157061683935));
#17932=CARTESIAN_POINT('Ctrl Pts',(6.32138714457423,-5.0672664088841,5.18795230177275));
#17933=CARTESIAN_POINT('Ctrl Pts',(6.80982170387704,-4.81064962531081,5.26294063889726));
#17934=CARTESIAN_POINT('Ctrl Pts',(7.17122043266886,-4.18554904460768,5.35628142326472));
#17935=CARTESIAN_POINT('Ctrl Pts',(6.97788741209539,-3.34365221835195,5.4675913947686));
#17936=CARTESIAN_POINT('Ctrl Pts',(6.38801757398717,-2.94404847700065,5.55969225114999));
#17937=CARTESIAN_POINT('Ctrl Pts',(5.84950720702512,-2.92590597485546,5.63294592890857));
#17938=CARTESIAN_POINT('Ctrl Pts',(5.42780119252992,-3.07275825516153,5.69374335618479));
#17939=CARTESIAN_POINT('Ctrl Pts',(5.07291053225168,-3.41926575125888,5.76029097754461));
#17940=CARTESIAN_POINT('Ctrl Pts',(4.91505669962947,-3.93339958881015,5.83246170467108));
#17941=CARTESIAN_POINT('Ctrl Pts',(5.00358120253044,-4.36965344538107,5.89223592257864));
#17942=CARTESIAN_POINT('Ctrl Pts',(5.16847877874769,-4.62410237756779,5.93387965098663));
#17943=CARTESIAN_POINT('Ctrl Pts',(5.28684674764252,-4.74851097849003,5.95761805778754));
#17944=CARTESIAN_POINT('Ctrl Pts',(5.48584905677489,-4.91159032288957,5.99316834802937));
#17945=CARTESIAN_POINT('Ctrl Pts',(5.85417679119542,-5.0558315382256,6.04627671719175));
#17946=CARTESIAN_POINT('Ctrl Pts',(6.33075428932811,-4.99570908084568,6.11075504563264));
#17947=CARTESIAN_POINT('Ctrl Pts',(6.69311737100275,-4.76738932049588,6.16902548955981));
#17948=CARTESIAN_POINT('Ctrl Pts',(6.92063937745368,-4.45890309164721,6.22119126264878));
#17949=CARTESIAN_POINT('Ctrl Pts',(7.01920463848466,-4.0904003195319,6.27308960467507));
#17950=CARTESIAN_POINT('Ctrl Pts',(6.97654392840764,-3.71341013806137,6.32471316097078));
#17951=CARTESIAN_POINT('Ctrl Pts',(6.79993515733336,-3.37991978141767,6.37606575989576));
#17952=CARTESIAN_POINT('Ctrl Pts',(6.51532665733549,-3.13506167065285,6.42714817101994));
#17953=CARTESIAN_POINT('Ctrl Pts',(6.16279711837762,-3.01213654187887,6.47796294003246));
#17954=CARTESIAN_POINT('Ctrl Pts',(5.72964410429838,-3.02816623710855,6.53693063505321));
#17955=CARTESIAN_POINT('Ctrl Pts',(5.28944670857787,-3.27117558494452,6.60389777235902));
#17956=CARTESIAN_POINT('Ctrl Pts',(5.0185771110185,-3.76349640673093,6.67865338334697));
#17957=CARTESIAN_POINT('Ctrl Pts',(5.04515925875904,-4.22673789405818,6.74047442293565));
#17958=CARTESIAN_POINT('Ctrl Pts',(5.21052884288523,-4.54528741933717,6.78966498160772));
#17959=CARTESIAN_POINT('Ctrl Pts',(5.41493563316234,-4.7617396587125,6.83050795551897));
#17960=CARTESIAN_POINT('Ctrl Pts',(5.70585879542675,-4.91537056653778,6.87525779471725));
#17961=CARTESIAN_POINT('Ctrl Pts',(6.06053583697364,-4.95510732388249,6.92384372352008));
#17962=CARTESIAN_POINT('Ctrl Pts',(6.46143918692318,-4.84800603500354,6.98028564004111));
#17963=CARTESIAN_POINT('Ctrl Pts',(6.82054812942106,-4.52694081115451,7.04444324737071));
#17964=CARTESIAN_POINT('Ctrl Pts',(6.96921975414278,-4.00847570947695,7.11621410834575));
#17965=CARTESIAN_POINT('Ctrl Pts',(6.82053287811316,-3.49368195718114,7.18758462714898));
#17966=CARTESIAN_POINT('Ctrl Pts',(6.42254980324896,-3.13829762703421,7.25860889560072));
#17967=CARTESIAN_POINT('Ctrl Pts',(5.89899472566348,-3.04994843752126,7.32930394453428));
#17968=CARTESIAN_POINT('Ctrl Pts',(5.4103834061862,-3.2524805765858,7.3997215654219));
#17969=CARTESIAN_POINT('Ctrl Pts',(5.10560112805102,-3.68264223188015,7.46990822314288));
#17970=CARTESIAN_POINT('Ctrl Pts',(5.07603810075024,-4.20761021857705,7.53991183200612));
#17971=CARTESIAN_POINT('Ctrl Pts',(5.33014059158489,-4.66688873918372,7.60978622792386));
#17972=CARTESIAN_POINT('Ctrl Pts',(5.7888549752637,-4.9203345943961,7.67956006945411));
#17973=CARTESIAN_POINT('Ctrl Pts',(6.31174238725869,-4.89093964456828,7.74928634435711));
#17974=CARTESIAN_POINT('Ctrl Pts',(6.73902593000717,-4.58796385083579,7.81901619775126));
#17975=CARTESIAN_POINT('Ctrl Pts',(6.93939676985519,-4.10372565119263,7.88878272235039));
#17976=CARTESIAN_POINT('Ctrl Pts',(6.851762373771,-3.58646485209147,7.95863747128128));
#17977=CARTESIAN_POINT('Ctrl Pts',(6.50145440276794,-3.1942196339742,8.02863622738192));
#17978=CARTESIAN_POINT('Ctrl Pts',(5.99506812255964,-3.04824066370828,8.09881519965856));
#17979=CARTESIAN_POINT('Ctrl Pts',(5.48652398303505,-3.19407539673001,8.16923214994343));
#17980=CARTESIAN_POINT('Ctrl Pts',(5.14580163911575,-3.57521396317503,8.23729514829861));
#17981=CARTESIAN_POINT('Ctrl Pts',(5.04892012023588,-4.0552555450462,8.30302386698914));
#17982=CARTESIAN_POINT('Ctrl Pts',(5.18740669602069,-4.50653622748511,8.36639189808384));
#17983=CARTESIAN_POINT('Ctrl Pts',(5.4986550261764,-4.81018052115883,8.42475683928535));
#17984=CARTESIAN_POINT('Ctrl Pts',(5.86844941776158,-4.93949335407164,8.4780524865146));
#17985=CARTESIAN_POINT('Ctrl Pts',(6.22215032474989,-4.9265097772033,8.52621674759037));
#17986=CARTESIAN_POINT('Ctrl Pts',(6.54798916354433,-4.7844123100289,8.57458080609539));
#17987=CARTESIAN_POINT('Ctrl Pts',(6.80055242150616,-4.53209565232151,8.62315924176611));
#17988=CARTESIAN_POINT('Ctrl Pts',(6.94413060607835,-4.2034339501668,8.67195830251317));
#17989=CARTESIAN_POINT('Ctrl Pts',(6.95777336420282,-3.84336797794748,8.72098623179676));
#17990=CARTESIAN_POINT('Ctrl Pts',(6.83835542549463,-3.50156151069008,8.77025013770849));
#17991=CARTESIAN_POINT('Ctrl Pts',(6.60115058604047,-3.22565815234949,8.81975670172189));
#17992=CARTESIAN_POINT('Ctrl Pts',(6.27792608816288,-3.05462702721105,8.86951191522505));
#17993=CARTESIAN_POINT('Ctrl Pts',(5.91269587682919,-3.01329689282491,8.91952105747049));
#17994=CARTESIAN_POINT('Ctrl Pts',(5.55577670770468,-3.10874082258239,8.96978893051619));
#17995=CARTESIAN_POINT('Ctrl Pts',(5.25682184453666,-3.32914518984797,9.02031918435157));
#17996=CARTESIAN_POINT('Ctrl Pts',(5.05804379683145,-3.6451580106137,9.07111583459068));
#17997=CARTESIAN_POINT('Ctrl Pts',(4.98800203972588,-4.01396234221588,9.12217980455873));
#17998=CARTESIAN_POINT('Ctrl Pts',(5.0580876534622,-4.38465341916386,9.17351671572958));
#17999=CARTESIAN_POINT('Ctrl Pts',(5.2819853526548,-4.74184810488963,9.23085986274571));
#18000=CARTESIAN_POINT('Ctrl Pts',(5.67872943927656,-4.99889438490076,9.29432501935413));
#18001=CARTESIAN_POINT('Ctrl Pts',(6.19695075641161,-5.03790457902352,9.36403899527298));
#18002=CARTESIAN_POINT('Ctrl Pts',(6.55940562763933,-4.87474206041059,9.41741918235656));
#18003=CARTESIAN_POINT('Ctrl Pts',(6.75506127473338,-4.69458762928485,9.45414031901828));
#18004=CARTESIAN_POINT('Ctrl Pts',(6.87668522837596,-4.54638877836258,9.48063024933242));
#18005=CARTESIAN_POINT('Ctrl Pts',(7.03301072347723,-4.245368303688,9.52711237127836));
#18006=CARTESIAN_POINT('Ctrl Pts',(7.06181762289588,-3.74471411884191,9.59388652174575));
#18007=CARTESIAN_POINT('Ctrl Pts',(6.7689591760146,-3.21363601446678,9.67459068366522));
#18008=CARTESIAN_POINT('Ctrl Pts',(6.23487010697712,-2.91779656590466,9.75585247155239));
#18009=CARTESIAN_POINT('Ctrl Pts',(5.62127050868205,-2.95181143891995,9.83765382096644));
#18010=CARTESIAN_POINT('Ctrl Pts',(5.11641195631316,-3.30899758881283,9.91996355293717));
#18011=CARTESIAN_POINT('Ctrl Pts',(4.87798505278271,-3.8836659287957,10.0027473525134));
#18012=CARTESIAN_POINT('Ctrl Pts',(4.98227272841176,-4.50036948740507,10.0859920067241));
#18013=CARTESIAN_POINT('Ctrl Pts',(5.40088585422602,-4.96944698093703,10.1696561496146));
#18014=CARTESIAN_POINT('Ctrl Pts',(6.00765739583399,-5.14465807361536,10.2537075984136));
#18015=CARTESIAN_POINT('Ctrl Pts',(6.61715595103273,-4.96943730503454,10.3381068322003));
#18016=CARTESIAN_POINT('Ctrl Pts',(7.04150787840671,-4.49504167195355,10.4228145333172));
#18017=CARTESIAN_POINT('Ctrl Pts',(7.14871630829242,-3.86560883063579,10.5077887784152));
#18018=CARTESIAN_POINT('Ctrl Pts',(6.90391357861512,-3.27408223567318,10.5929860562277));
#18019=CARTESIAN_POINT('Ctrl Pts',(6.38081263394418,-2.90272063471259,10.6783623214699));
#18020=CARTESIAN_POINT('Ctrl Pts',(5.73926233026402,-2.86658474978731,10.7638702346137));
#18021=CARTESIAN_POINT('Ctrl Pts',(5.17635857755646,-3.17764139675116,10.849466654309));
#18022=CARTESIAN_POINT('Ctrl Pts',(4.86489677958424,-3.74082925476046,10.9350964140044));
#18023=CARTESIAN_POINT('Ctrl Pts',(4.90133545189447,-4.383198400959,11.0207291628158));
#18024=CARTESIAN_POINT('Ctrl Pts',(5.27331123911313,-4.90761852821718,11.1063112487012));
#18025=CARTESIAN_POINT('Ctrl Pts',(5.8667411442123,-5.15320882638912,11.1917885764413));
#18026=CARTESIAN_POINT('Ctrl Pts',(6.49868316645557,-5.0458533596991,11.2771194094233));
#18027=CARTESIAN_POINT('Ctrl Pts',(6.97547246984522,-4.61907226633235,11.3622555926326));
#18028=CARTESIAN_POINT('Ctrl Pts',(7.09288943197313,-4.21115651665385,11.4188571787892));
#18029=CARTESIAN_POINT('Ctrl Pts',(7.09291698096071,-4.0065158743674,11.4471081759743));
#18030=CARTESIAN_POINT('Ctrl Pts',(6.91041388003776,-3.99025785493753,2.62934384528526));
#18031=CARTESIAN_POINT('Ctrl Pts',(6.91039080704782,-3.81886569155907,2.65300483199757));
#18032=CARTESIAN_POINT('Ctrl Pts',(6.8122491622858,-3.47775408576118,2.70033480637834));
#18033=CARTESIAN_POINT('Ctrl Pts',(6.41196409991056,-3.11888567055589,2.77187288605298));
#18034=CARTESIAN_POINT('Ctrl Pts',(5.87870459195709,-3.02800305041287,2.84387354450334));
#18035=CARTESIAN_POINT('Ctrl Pts',(5.37501897776042,-3.23595938105673,2.91641672576983));
#18036=CARTESIAN_POINT('Ctrl Pts',(5.05670377179691,-3.68359061413889,2.98951226441559));
#18037=CARTESIAN_POINT('Ctrl Pts',(5.02516628278399,-4.23620154296935,3.06319721265735));
#18038=CARTESIAN_POINT('Ctrl Pts',(5.29433269147969,-4.72517576991202,3.13748867038598));
#18039=CARTESIAN_POINT('Ctrl Pts',(5.78679871047612,-4.99797595495716,3.21240611140967));
#18040=CARTESIAN_POINT('Ctrl Pts',(6.35363537824581,-4.96685750155159,3.28797094288595));
#18041=CARTESIAN_POINT('Ctrl Pts',(6.8211198508534,-4.63603041178032,3.36419307761376));
#18042=CARTESIAN_POINT('Ctrl Pts',(7.04283368983127,-4.10260934326042,3.4410820879014));
#18043=CARTESIAN_POINT('Ctrl Pts',(6.94594187284151,-3.52801981043285,3.51864207258902));
#18044=CARTESIAN_POINT('Ctrl Pts',(6.55482388157473,-3.08929256377072,3.59687389466955));
#18045=CARTESIAN_POINT('Ctrl Pts',(5.98544482856865,-2.92453923112812,3.67577412964314));
#18046=CARTESIAN_POINT('Ctrl Pts',(5.41085897745953,-3.08930968376791,3.75533558541602));
#18047=CARTESIAN_POINT('Ctrl Pts',(5.02379505335764,-3.52165808238205,3.83257622804987));
#18048=CARTESIAN_POINT('Ctrl Pts',(4.931020522875,-3.98066380798232,3.89542943544965));
#18049=CARTESIAN_POINT('Ctrl Pts',(4.9844408484075,-4.28254645693087,3.93754525316638));
#18050=CARTESIAN_POINT('Ctrl Pts',(5.04619135722488,-4.44582563834565,3.96167148603502));
#18051=CARTESIAN_POINT('Ctrl Pts',(5.16861301581523,-4.67780809698434,3.99792049351659));
#18052=CARTESIAN_POINT('Ctrl Pts',(5.45946253135908,-4.96217671243346,4.05251748479476));
#18053=CARTESIAN_POINT('Ctrl Pts',(5.98468607065537,-5.11036489028024,4.12576694910513));
#18054=CARTESIAN_POINT('Ctrl Pts',(6.52011973324497,-4.98866785198386,4.19945297410707));
#18055=CARTESIAN_POINT('Ctrl Pts',(6.89945162846597,-4.65370085290913,4.26738008926097));
#18056=CARTESIAN_POINT('Ctrl Pts',(7.08165637686814,-4.23578697094255,4.32941453727684));
#18057=CARTESIAN_POINT('Ctrl Pts',(7.09743152418886,-3.82420346898175,4.38545624718568));
#18058=CARTESIAN_POINT('Ctrl Pts',(6.96082001314597,-3.43420568070724,4.44169499055966));
#18059=CARTESIAN_POINT('Ctrl Pts',(6.66069499579344,-3.08446880580411,4.50439011816686));
#18060=CARTESIAN_POINT('Ctrl Pts',(6.19086806115881,-2.87223085510411,4.5736016912126));
#18061=CARTESIAN_POINT('Ctrl Pts',(5.62770576916625,-2.91422420562986,4.64938324638858));
#18062=CARTESIAN_POINT('Ctrl Pts',(5.25111785199374,-3.15750274058377,4.70958190751128));
#18063=CARTESIAN_POINT('Ctrl Pts',(5.05509817427152,-3.41339807779548,4.75401872379404));
#18064=CARTESIAN_POINT('Ctrl Pts',(4.93029391983906,-3.66017056351555,4.79214573005493));
#18065=CARTESIAN_POINT('Ctrl Pts',(4.86499221929501,-4.0048010675327,4.83987165496948));
#18066=CARTESIAN_POINT('Ctrl Pts',(4.94344411857747,-4.41899208362928,4.89723533807431));
#18067=CARTESIAN_POINT('Ctrl Pts',(5.16791520878115,-4.77657053811553,4.954677607837));
#18068=CARTESIAN_POINT('Ctrl Pts',(5.50792791889865,-5.02736403777264,5.01218255346116));
#18069=CARTESIAN_POINT('Ctrl Pts',(5.91660949347755,-5.13715603053052,5.06973457806084));
#18070=CARTESIAN_POINT('Ctrl Pts',(6.3367779644244,-5.08942543737139,5.12731888318447));
#18071=CARTESIAN_POINT('Ctrl Pts',(6.83702927977863,-4.82679209842469,5.20411951082081));
#18072=CARTESIAN_POINT('Ctrl Pts',(7.20933766937117,-4.18431587015626,5.30013430054567));
#18073=CARTESIAN_POINT('Ctrl Pts',(7.01034570705962,-3.31366155048617,5.41523225831058));
#18074=CARTESIAN_POINT('Ctrl Pts',(6.3977364131714,-2.89784267685387,5.5109554305934));
#18075=CARTESIAN_POINT('Ctrl Pts',(5.83613927351209,-2.87878248811417,5.58735163070686));
#18076=CARTESIAN_POINT('Ctrl Pts',(5.39535814415608,-3.03217873181673,5.65090114175908));
#18077=CARTESIAN_POINT('Ctrl Pts',(5.02334729005529,-3.3951294460668,5.72063905656003));
#18078=CARTESIAN_POINT('Ctrl Pts',(4.85728925835324,-3.93530401284747,5.79647914846814));
#18079=CARTESIAN_POINT('Ctrl Pts',(4.95040053000959,-4.3948784892822,5.85944685621913));
#18080=CARTESIAN_POINT('Ctrl Pts',(5.12438570171492,-4.66340933665913,5.90339414657583));
#18081=CARTESIAN_POINT('Ctrl Pts',(5.2493935187274,-4.79480118236336,5.92846496633277));
#18082=CARTESIAN_POINT('Ctrl Pts',(5.4596703719434,-4.96713107722029,5.96603147351556));
#18083=CARTESIAN_POINT('Ctrl Pts',(5.8493603739367,-5.11985609810124,6.02222723777501));
#18084=CARTESIAN_POINT('Ctrl Pts',(6.35460113952391,-5.05624174985086,6.09058222260399));
#18085=CARTESIAN_POINT('Ctrl Pts',(6.73933984369154,-4.81390063965477,6.15244556102042));
#18086=CARTESIAN_POINT('Ctrl Pts',(6.98118457887927,-4.48606318884047,6.20788769925023));
#18087=CARTESIAN_POINT('Ctrl Pts',(7.08608186634963,-4.09405409466647,6.26309751878246));
#18088=CARTESIAN_POINT('Ctrl Pts',(7.04069467998163,-3.69267509562981,6.31805903401915));
#18089=CARTESIAN_POINT('Ctrl Pts',(6.85256366464928,-3.33737104537872,6.3727674879457));
#18090=CARTESIAN_POINT('Ctrl Pts',(6.54921482208544,-3.07635812326129,6.42721377541));
#18091=CARTESIAN_POINT('Ctrl Pts',(6.17333370611417,-2.94527448076034,6.48139220696859));
#18092=CARTESIAN_POINT('Ctrl Pts',(5.71139634990446,-2.96235904620064,6.54427642819304));
#18093=CARTESIAN_POINT('Ctrl Pts',(5.24195855587125,-3.22150171333028,6.61568196044263));
#18094=CARTESIAN_POINT('Ctrl Pts',(4.95324402611607,-3.74634709443177,6.69536386654557));
#18095=CARTESIAN_POINT('Ctrl Pts',(4.98161750117062,-4.23980174957217,6.76121320872448));
#18096=CARTESIAN_POINT('Ctrl Pts',(5.15763242426064,-4.57881842470844,6.81356023789864));
#18097=CARTESIAN_POINT('Ctrl Pts',(5.37504268972789,-4.80902468214805,6.85699616204033));
#18098=CARTESIAN_POINT('Ctrl Pts',(5.68418613989248,-4.97223633786759,6.90453778880486));
#18099=CARTESIAN_POINT('Ctrl Pts',(6.06062183697248,-5.01436815416344,6.95610098888784));
#18100=CARTESIAN_POINT('Ctrl Pts',(6.48550711521371,-4.90080029315905,7.01591156763435));
#18101=CARTESIAN_POINT('Ctrl Pts',(6.86525409936937,-4.56104588973726,7.08377161093949));
#18102=CARTESIAN_POINT('Ctrl Pts',(7.02186082581237,-4.01409341078421,7.15945586805767));
#18103=CARTESIAN_POINT('Ctrl Pts',(6.86526232149639,-3.47282042782154,7.23449212322981));
#18104=CARTESIAN_POINT('Ctrl Pts',(6.44802413959838,-3.10062213493182,7.30889612256709));
#18105=CARTESIAN_POINT('Ctrl Pts',(5.901400424226,-3.00870277543536,7.3826878474804));
#18106=CARTESIAN_POINT('Ctrl Pts',(5.39352039285457,-3.21957437439377,7.45588985731414));
#18107=CARTESIAN_POINT('Ctrl Pts',(5.07833615802819,-3.66503206095406,7.5285291186389));
#18108=CARTESIAN_POINT('Ctrl Pts',(5.04823664994393,-4.20588633168366,7.60063427930656));
#18109=CARTESIAN_POINT('Ctrl Pts',(5.30904925496711,-4.67648866522258,7.67223726675353));
#18110=CARTESIAN_POINT('Ctrl Pts',(5.77705173780209,-4.93462323268497,7.74337645487925));
#18111=CARTESIAN_POINT('Ctrl Pts',(6.30746620650405,-4.90439550306326,7.81409007533856));
#18112=CARTESIAN_POINT('Ctrl Pts',(6.73832012465397,-4.598388527706,7.88441740191195));
#18113=CARTESIAN_POINT('Ctrl Pts',(6.93898456949613,-4.11235148307006,7.95440671960687));
#18114=CARTESIAN_POINT('Ctrl Pts',(6.85113932402579,-3.59626983255766,8.02410221512531));
#18115=CARTESIAN_POINT('Ctrl Pts',(6.50323102966143,-3.20732217322844,8.09354734997649));
#18116=CARTESIAN_POINT('Ctrl Pts',(6.00339991092543,-3.06365063168461,8.16279549808777));
#18117=CARTESIAN_POINT('Ctrl Pts',(5.50439671438939,-3.20715934459842,8.23188849529843));
#18118=CARTESIAN_POINT('Ctrl Pts',(5.17202190935144,-3.57951563299814,8.29833266947451));
#18119=CARTESIAN_POINT('Ctrl Pts',(5.07818019990084,-4.04593165133975,8.36217277635728));
#18120=CARTESIAN_POINT('Ctrl Pts',(5.21238143820554,-4.48240836001952,8.42346320100455));
#18121=CARTESIAN_POINT('Ctrl Pts',(5.51236025777204,-4.77474404476563,8.47967815909619));
#18122=CARTESIAN_POINT('Ctrl Pts',(5.86737823061201,-4.89877834106162,8.53083636744996));
#18123=CARTESIAN_POINT('Ctrl Pts',(6.20593010073297,-4.88625474217651,8.57692807693114));
#18124=CARTESIAN_POINT('Ctrl Pts',(6.5169557998887,-4.75052124336708,8.62309627990358));
#18125=CARTESIAN_POINT('Ctrl Pts',(6.75738085499608,-4.51021173196975,8.66934525439234));
#18126=CARTESIAN_POINT('Ctrl Pts',(6.89369213325771,-4.19798398918876,8.71569439753526));
#18127=CARTESIAN_POINT('Ctrl Pts',(6.90654691277405,-3.85671872643878,8.76215710981506));
#18128=CARTESIAN_POINT('Ctrl Pts',(6.79353247440965,-3.53345392369584,8.80874771009088));
#18129=CARTESIAN_POINT('Ctrl Pts',(6.56955414486768,-3.27303442323799,8.85547967409816));
#18130=CARTESIAN_POINT('Ctrl Pts',(6.2649149706205,-3.11190453193631,8.90236637798983));
#18131=CARTESIAN_POINT('Ctrl Pts',(5.92123870946621,-3.07306727004794,8.94942058038104));
#18132=CARTESIAN_POINT('Ctrl Pts',(5.58585464057643,-3.16280189459015,8.99665488281507));
#18133=CARTESIAN_POINT('Ctrl Pts',(5.30528004465418,-3.36970780699163,9.04408084976179));
#18134=CARTESIAN_POINT('Ctrl Pts',(5.11891923625802,-3.66604749262102,9.09171075577402));
#18135=CARTESIAN_POINT('Ctrl Pts',(5.05332609200974,-4.01160086184926,9.13955361060455));
#18136=CARTESIAN_POINT('Ctrl Pts',(5.1189740076943,-4.35870259389239,9.18762398931142));
#18137=CARTESIAN_POINT('Ctrl Pts',(5.3285542005314,-4.6930196813579,9.24129614057046));
#18138=CARTESIAN_POINT('Ctrl Pts',(5.6998052948892,-4.93352876813364,9.30068292152737));
#18139=CARTESIAN_POINT('Ctrl Pts',(6.18472180410833,-4.97003234438759,9.36591862472348));
#18140=CARTESIAN_POINT('Ctrl Pts',(6.52399659312322,-4.81732094542808,9.41588571108487));
#18141=CARTESIAN_POINT('Ctrl Pts',(6.7072097546456,-4.64862385300487,9.45027233971667));
#18142=CARTESIAN_POINT('Ctrl Pts',(6.82112063385224,-4.50982226066863,9.47508293238151));
#18143=CARTESIAN_POINT('Ctrl Pts',(6.96758616721527,-4.2277942769692,9.51863575059301));
#18144=CARTESIAN_POINT('Ctrl Pts',(6.99467197393324,-3.7583480064713,9.5812519512241));
#18145=CARTESIAN_POINT('Ctrl Pts',(6.7197786782019,-3.25958856827978,9.65704089928746));
#18146=CARTESIAN_POINT('Ctrl Pts',(6.21742976902802,-2.98115434624709,9.73349110143862));
#18147=CARTESIAN_POINT('Ctrl Pts',(5.63898185512583,-3.01303591196271,9.81061012778847));
#18148=CARTESIAN_POINT('Ctrl Pts',(5.16178296910393,-3.3504033680704,9.88840029758739));
#18149=CARTESIAN_POINT('Ctrl Pts',(4.93563437526279,-3.89485977010871,9.9668597654298));
#18150=CARTESIAN_POINT('Ctrl Pts',(5.03449733338635,-4.48101061407005,10.0459867177188));
#18151=CARTESIAN_POINT('Ctrl Pts',(5.43341655784522,-4.92844358267535,10.1257712061144));
#18152=CARTESIAN_POINT('Ctrl Pts',(6.01386261401897,-5.09636465569706,10.2062013199047));
#18153=CARTESIAN_POINT('Ctrl Pts',(6.599221886597,-4.92841521164529,10.2872604826976));
#18154=CARTESIAN_POINT('Ctrl Pts',(7.00852275003305,-4.47134999264525,10.3689288213763));
#18155=CARTESIAN_POINT('Ctrl Pts',(7.11262626892049,-3.86224370688857,10.451182632454));
#18156=CARTESIAN_POINT('Ctrl Pts',(6.87506262144489,-3.28725204329248,10.5339950246611));
#18157=CARTESIAN_POINT('Ctrl Pts',(6.36475855714357,-2.92451218932454,10.6173353554807));
#18158=CARTESIAN_POINT('Ctrl Pts',(5.7359246081994,-2.88870804221006,10.7011708628368));
#18159=CARTESIAN_POINT('Ctrl Pts',(5.18151714958306,-3.19462123968635,10.785463758442));
#18160=CARTESIAN_POINT('Ctrl Pts',(4.87313525619405,-3.75143465324639,10.8701783685472));
#18161=CARTESIAN_POINT('Ctrl Pts',(4.90893297033217,-4.3896485385702,10.9552659908788));
#18162=CARTESIAN_POINT('Ctrl Pts',(5.27984440785336,-4.91323561648797,11.0406883269263));
#18163=CARTESIAN_POINT('Ctrl Pts',(5.87465010049056,-5.15984481059548,11.1263952635579));
#18164=CARTESIAN_POINT('Ctrl Pts',(6.51118263329733,-5.05207927242605,11.212352848697));
#18165=CARTESIAN_POINT('Ctrl Pts',(6.99381915840408,-4.62071977485365,11.2984788432175));
#18166=CARTESIAN_POINT('Ctrl Pts',(7.11344761293339,-4.20611912793284,11.3560318805412));
#18167=CARTESIAN_POINT('Ctrl Pts',(7.11347564185152,-3.99791344370584,11.3847750379771));
#18168=CARTESIAN_POINT('Ctrl Pts',(6.88853642595183,-4.00349313356656,2.72519438129392));
#18169=CARTESIAN_POINT('Ctrl Pts',(6.88851392453586,-3.83634677012002,2.74826922792962));
#18170=CARTESIAN_POINT('Ctrl Pts',(6.79266191595664,-3.50459201237406,2.79432671715279));
#18171=CARTESIAN_POINT('Ctrl Pts',(6.40607867092915,-3.15886656679987,2.86334141911335));
#18172=CARTESIAN_POINT('Ctrl Pts',(5.89537108171216,-3.07233178035552,2.93229916216477));
#18173=CARTESIAN_POINT('Ctrl Pts',(5.41675202428946,-3.27049076436878,3.0012653898671));
#18174=CARTESIAN_POINT('Ctrl Pts',(5.11661138750114,-3.69336572084077,3.07028597393075));
#18175=CARTESIAN_POINT('Ctrl Pts',(5.08746128376669,-4.21176251067231,3.13941287767591));
#18176=CARTESIAN_POINT('Ctrl Pts',(5.33882111712877,-4.66753429258786,3.20869886998172));
#18177=CARTESIAN_POINT('Ctrl Pts',(5.7957396457742,-4.92022616783295,3.27819757081899));
#18178=CARTESIAN_POINT('Ctrl Pts',(6.31886968522155,-4.89117427234567,3.34794867589613));
#18179=CARTESIAN_POINT('Ctrl Pts',(6.74829250702319,-4.58692636184723,3.41800335411985));
#18180=CARTESIAN_POINT('Ctrl Pts',(6.95104349855107,-4.09847642990215,3.48840505118448));
#18181=CARTESIAN_POINT('Ctrl Pts',(6.86241194209975,-3.57411489808785,3.55919775533007));
#18182=CARTESIAN_POINT('Ctrl Pts',(6.50624110521479,-3.17483224994897,3.63042194356993));
#18183=CARTESIAN_POINT('Ctrl Pts',(5.98887372723457,-3.02524962710709,3.70211601317391));
#18184=CARTESIAN_POINT('Ctrl Pts',(5.46750934114836,-3.17483111712725,3.77431546014986));
#18185=CARTESIAN_POINT('Ctrl Pts',(5.11654649260021,-3.56688533544979,3.84435869757401));
#18186=CARTESIAN_POINT('Ctrl Pts',(5.03241283783216,-3.98305413265401,3.90134876203804));
#18187=CARTESIAN_POINT('Ctrl Pts',(5.08085289836134,-4.25684105267147,3.93954512081593));
#18188=CARTESIAN_POINT('Ctrl Pts',(5.13686700531774,-4.40495648433533,3.96143070534772));
#18189=CARTESIAN_POINT('Ctrl Pts',(5.24793660806346,-4.61543096030812,3.99431888928194));
#18190=CARTESIAN_POINT('Ctrl Pts',(5.51191441648992,-4.87360832231182,4.04387894827305));
#18191=CARTESIAN_POINT('Ctrl Pts',(5.98925640546539,-5.00838455128162,4.11045355448925));
#18192=CARTESIAN_POINT('Ctrl Pts',(6.47674305919525,-4.8977142557422,4.17753674404586));
#18193=CARTESIAN_POINT('Ctrl Pts',(6.82290576508146,-4.59223022955248,4.23950296796532));
#18194=CARTESIAN_POINT('Ctrl Pts',(6.98956599692813,-4.21016952566571,4.29621883871687));
#18195=CARTESIAN_POINT('Ctrl Pts',(7.00410282218404,-3.83310156474722,4.34755879606028));
#18196=CARTESIAN_POINT('Ctrl Pts',(6.87874007455572,-3.47495996875609,4.39919719455462));
#18197=CARTESIAN_POINT('Ctrl Pts',(6.60256885276253,-3.15296728990473,4.45690377989833));
#18198=CARTESIAN_POINT('Ctrl Pts',(6.16884895912283,-2.95679731990753,4.52080650172853));
#18199=CARTESIAN_POINT('Ctrl Pts',(5.64683817264842,-2.99545349895525,4.59104572930851));
#18200=CARTESIAN_POINT('Ctrl Pts',(5.29623798334719,-3.22166642760234,4.64705739245952));
#18201=CARTESIAN_POINT('Ctrl Pts',(5.11321685115952,-3.46054845990971,4.6885396246491));
#18202=CARTESIAN_POINT('Ctrl Pts',(4.99649312835915,-3.69129778885919,4.72419099996777));
#18203=CARTESIAN_POINT('Ctrl Pts',(4.93515842947507,-4.01438075257337,4.76893235210618));
#18204=CARTESIAN_POINT('Ctrl Pts',(5.00884138794006,-4.40411676050145,4.82290104831588));
#18205=CARTESIAN_POINT('Ctrl Pts',(5.22069691149792,-4.74188211024749,4.87714211347641));
#18206=CARTESIAN_POINT('Ctrl Pts',(5.54294475281331,-4.979743888843,4.93165037763781));
#18207=CARTESIAN_POINT('Ctrl Pts',(5.93184914211983,-5.08439121416751,4.98641884848078));
#18208=CARTESIAN_POINT('Ctrl Pts',(6.33337868619195,-5.03891906119859,5.04143962102492));
#18209=CARTESIAN_POINT('Ctrl Pts',(6.81344622817293,-4.78714604268289,5.11512659410201));
#18210=CARTESIAN_POINT('Ctrl Pts',(7.17386284388877,-4.16740765547856,5.20781208817404));
#18211=CARTESIAN_POINT('Ctrl Pts',(6.98151177291868,-3.31910065636828,5.31989742715281));
#18212=CARTESIAN_POINT('Ctrl Pts',(6.38018037258757,-2.90949829895718,5.41393652817617));
#18213=CARTESIAN_POINT('Ctrl Pts',(5.82452419881361,-2.89038561056404,5.4895085736308));
#18214=CARTESIAN_POINT('Ctrl Pts',(5.38643937700961,-3.0426430278763,5.55265631890358));
#18215=CARTESIAN_POINT('Ctrl Pts',(5.0145022718477,-3.40495936093987,5.62231958033395));
#18216=CARTESIAN_POINT('Ctrl Pts',(4.84717711780572,-3.94776217453295,5.69853006603046));
#18217=CARTESIAN_POINT('Ctrl Pts',(4.94099186919954,-4.41256002942381,5.76219880693713));
#18218=CARTESIAN_POINT('Ctrl Pts',(5.11766856031632,-4.68536215086932,5.80682961590476));
#18219=CARTESIAN_POINT('Ctrl Pts',(5.24493119859604,-4.81913238240527,5.83235224216694));
#18220=CARTESIAN_POINT('Ctrl Pts',(5.45930477431542,-4.9948414663518,5.87065055301519));
#18221=CARTESIAN_POINT('Ctrl Pts',(5.85797322925551,-5.15141705336824,5.92814987557556));
#18222=CARTESIAN_POINT('Ctrl Pts',(6.37807174974638,-5.08631909572604,5.99849836625092));
#18223=CARTESIAN_POINT('Ctrl Pts',(6.77618145548473,-4.83577308391186,6.06247866417908));
#18224=CARTESIAN_POINT('Ctrl Pts',(7.02758555630676,-4.49525125160203,6.12008054118587));
#18225=CARTESIAN_POINT('Ctrl Pts',(7.13717722861579,-4.08632109309765,6.1776704930539));
#18226=CARTESIAN_POINT('Ctrl Pts',(7.08979000943633,-3.66582201155788,6.23524265529162));
#18227=CARTESIAN_POINT('Ctrl Pts',(6.89204673042122,-3.29205056628206,6.29277697865426));
#18228=CARTESIAN_POINT('Ctrl Pts',(6.5718504683246,-3.01633590404546,6.35026012152877));
#18229=CARTESIAN_POINT('Ctrl Pts',(6.17349702418284,-2.87727195418905,6.40767537367819));
#18230=CARTESIAN_POINT('Ctrl Pts',(5.68208662701439,-2.89527617243405,6.47456940039547));
#18231=CARTESIAN_POINT('Ctrl Pts',(5.18032599444233,-3.17179956913016,6.55085081859633));
#18232=CARTESIAN_POINT('Ctrl Pts',(4.86989550108574,-3.73521723461931,6.63640620982512));
#18233=CARTESIAN_POINT('Ctrl Pts',(4.90018724897131,-4.26763558163364,6.70744811984369));
#18234=CARTESIAN_POINT('Ctrl Pts',(5.09065881531276,-4.6346219832112,6.76410197014731));
#18235=CARTESIAN_POINT('Ctrl Pts',(5.32642853144266,-4.88432892504754,6.81120999936015));
#18236=CARTESIAN_POINT('Ctrl Pts',(5.66244422861094,-5.06182402697993,6.86288433937329));
#18237=CARTESIAN_POINT('Ctrl Pts',(6.07263963889414,-5.10781715858294,6.91907132462124));
#18238=CARTESIAN_POINT('Ctrl Pts',(6.53667667508948,-4.98388363300407,6.98438658115342));
#18239=CARTESIAN_POINT('Ctrl Pts',(6.95258347663703,-4.61205745986084,7.05868174802314));
#18240=CARTESIAN_POINT('Ctrl Pts',(7.12466537226074,-4.01175995341158,7.14174808909433));
#18241=CARTESIAN_POINT('Ctrl Pts',(6.95256249513245,-3.41639873131959,7.22427322871735));
#18242=CARTESIAN_POINT('Ctrl Pts',(6.49303513416945,-3.00635077992184,7.30622569076459));
#18243=CARTESIAN_POINT('Ctrl Pts',(5.89035880333171,-2.90495807984544,7.38758293290033));
#18244=CARTESIAN_POINT('Ctrl Pts',(5.33018372919521,-3.13754016396607,7.46832214054757));
#18245=CARTESIAN_POINT('Ctrl Pts',(4.98265794015465,-3.62878963133895,7.54842402890944));
#18246=CARTESIAN_POINT('Ctrl Pts',(4.94959218817397,-4.22473472744915,7.62787515983858));
#18247=CARTESIAN_POINT('Ctrl Pts',(5.23670236553316,-4.74246459176775,7.7066648962458));
#18248=CARTESIAN_POINT('Ctrl Pts',(5.75070331377736,-5.02573461363327,7.78478658453007));
#18249=CARTESIAN_POINT('Ctrl Pts',(6.3315944612577,-4.99238023588094,7.86223715968712));
#18250=CARTESIAN_POINT('Ctrl Pts',(6.80176712773346,-4.65807183999786,7.93901966146638));
#18251=CARTESIAN_POINT('Ctrl Pts',(7.01966294687514,-4.12940487515114,8.01513582983289));
#18252=CARTESIAN_POINT('Ctrl Pts',(6.92418292551131,-3.57072879727912,8.09059580794518));
#18253=CARTESIAN_POINT('Ctrl Pts',(6.54906751855537,-3.15201220927634,8.16541569688595));
#18254=CARTESIAN_POINT('Ctrl Pts',(6.01345996886975,-2.99852359627092,8.23960831004383));
#18255=CARTESIAN_POINT('Ctrl Pts',(5.48217439877857,-3.15184573564912,8.31320179685831));
#18256=CARTESIAN_POINT('Ctrl Pts',(5.13089843772479,-3.54612521955196,8.38350581076996));
#18257=CARTESIAN_POINT('Ctrl Pts',(5.0326487563089,-4.0364884839662,8.45062953683967));
#18258=CARTESIAN_POINT('Ctrl Pts',(5.17319067664245,-4.49223316217463,8.51464838787996));
#18259=CARTESIAN_POINT('Ctrl Pts',(5.48463728440744,-4.79523144276229,8.5729734529706));
#18260=CARTESIAN_POINT('Ctrl Pts',(5.85075368554384,-4.92293243199514,8.62572747369152));
#18261=CARTESIAN_POINT('Ctrl Pts',(6.19801348687623,-4.90991155246289,8.67301780183671));
#18262=CARTESIAN_POINT('Ctrl Pts',(6.51522255886468,-4.77128712747284,8.72011840453903));
#18263=CARTESIAN_POINT('Ctrl Pts',(6.75903612701758,-4.52733816748863,8.76705321549295));
#18264=CARTESIAN_POINT('Ctrl Pts',(6.89641433024893,-4.21221927191064,8.81382959040646));
#18265=CARTESIAN_POINT('Ctrl Pts',(6.90913619885495,-3.86977043889933,8.86046173222151));
#18266=CARTESIAN_POINT('Ctrl Pts',(6.79619374111234,-3.54724787641334,8.90696283891172));
#18267=CARTESIAN_POINT('Ctrl Pts',(6.57379330446791,-3.28893297442313,8.95334702636426));
#18268=CARTESIAN_POINT('Ctrl Pts',(6.27306517518208,-3.13006968654134,8.99962841810225));
#18269=CARTESIAN_POINT('Ctrl Pts',(5.93572658739197,-3.0921235656841,9.0458216557526));
#18270=CARTESIAN_POINT('Ctrl Pts',(5.60836618975707,-3.17988842208988,9.09194124619793));
#18271=CARTESIAN_POINT('Ctrl Pts',(5.33602236999747,-3.38093608109373,9.13800263745416));
#18272=CARTESIAN_POINT('Ctrl Pts',(5.15614240909104,-3.66727534380435,9.18401982014308));
#18273=CARTESIAN_POINT('Ctrl Pts',(5.09326323380394,-3.99940669517924,9.23001051026176));
#18274=CARTESIAN_POINT('Ctrl Pts',(5.15618727724121,-4.33129335464849,9.27598439739637));
#18275=CARTESIAN_POINT('Ctrl Pts',(5.35578605418237,-4.64936719014534,9.32706877285428));
#18276=CARTESIAN_POINT('Ctrl Pts',(5.70736198634476,-4.87675366561928,9.3832866314104));
#18277=CARTESIAN_POINT('Ctrl Pts',(6.16369266354364,-4.91077958536555,9.44468658180074));
#18278=CARTESIAN_POINT('Ctrl Pts',(6.48109710311922,-4.76766612382848,9.49145069598086));
#18279=CARTESIAN_POINT('Ctrl Pts',(6.65197106906924,-4.61031651982011,9.52352657457864));
#18280=CARTESIAN_POINT('Ctrl Pts',(6.75806246750007,-4.48103427992951,9.54663607519105));
#18281=CARTESIAN_POINT('Ctrl Pts',(6.89415792745756,-4.21884193757629,9.58712522676296));
#18282=CARTESIAN_POINT('Ctrl Pts',(6.91894087007071,-3.78418172620761,9.64510513260814));
#18283=CARTESIAN_POINT('Ctrl Pts',(6.66534324481484,-3.32472290943998,9.71495345065709));
#18284=CARTESIAN_POINT('Ctrl Pts',(6.20419942989133,-3.06944166542164,9.78511977938196));
#18285=CARTESIAN_POINT('Ctrl Pts',(5.67524333022435,-3.09882568028089,9.85564775939405));
#18286=CARTESIAN_POINT('Ctrl Pts',(5.24024568965602,-3.40659380896812,9.92658189146111));
#18287=CARTESIAN_POINT('Ctrl Pts',(5.03464763548414,-3.90193118025057,9.99796464537582));
#18288=CARTESIAN_POINT('Ctrl Pts',(5.12452333571866,-4.43421378319489,10.0698272337774));
#18289=CARTESIAN_POINT('Ctrl Pts',(5.48642962474464,-4.84005659450095,10.1422070537588));
#18290=CARTESIAN_POINT('Ctrl Pts',(6.01270459980476,-4.99229906382123,10.2151342966527));
#18291=CARTESIAN_POINT('Ctrl Pts',(6.54349151359531,-4.84004652702854,10.2886377190555));
#18292=CARTESIAN_POINT('Ctrl Pts',(6.91493654437396,-4.42537746826921,10.3627418267029));
#18293=CARTESIAN_POINT('Ctrl Pts',(7.00963644867476,-3.87203813765055,10.4374679148733));
#18294=CARTESIAN_POINT('Ctrl Pts',(6.79358830396164,-3.34867882889457,10.5128334140703));
#18295=CARTESIAN_POINT('Ctrl Pts',(6.32822477073631,-3.01762364049853,10.5888520780036));
#18296=CARTESIAN_POINT('Ctrl Pts',(5.75303331970575,-2.98461572568303,10.665533657142));
#18297=CARTESIAN_POINT('Ctrl Pts',(5.24411579401217,-3.26509167414394,10.7428842026003));
#18298=CARTESIAN_POINT('Ctrl Pts',(4.95977091463743,-3.77778621479579,10.8209053147198));
#18299=CARTESIAN_POINT('Ctrl Pts',(4.99250844096273,-4.36807972196266,10.8995957097798));
#18300=CARTESIAN_POINT('Ctrl Pts',(5.33676307768738,-4.85473515789548,10.9789525208368));
#18301=CARTESIAN_POINT('Ctrl Pts',(5.89185847419169,-5.0853624635031,11.0589565134979));
#18302=CARTESIAN_POINT('Ctrl Pts',(6.48921656678778,-4.98467525931286,11.1396133726823));
#18303=CARTESIAN_POINT('Ctrl Pts',(6.94489938062386,-4.57808986983126,11.2208627112899));
#18304=CARTESIAN_POINT('Ctrl Pts',(7.05869952443909,-4.18467099703403,11.2754820789842));
#18305=CARTESIAN_POINT('Ctrl Pts',(7.05872618995271,-3.98659301618569,11.3028270893246));
#18306=CARTESIAN_POINT('Ctrl Pts',(6.95029270794106,-4.01413412167565,2.80233431196407));
#18307=CARTESIAN_POINT('Ctrl Pts',(6.95026870797549,-3.83585614248054,2.82694589754466));
#18308=CARTESIAN_POINT('Ctrl Pts',(6.84793152004367,-3.48237875324069,2.87602065146748));
#18309=CARTESIAN_POINT('Ctrl Pts',(6.43858029515218,-3.11708365014168,2.94901647539155));
#18310=CARTESIAN_POINT('Ctrl Pts',(5.90189353794577,-3.02662837560554,3.02147175614449));
#18311=CARTESIAN_POINT('Ctrl Pts',(5.40287867078653,-3.23386954835159,3.09339843495734));
#18312=CARTESIAN_POINT('Ctrl Pts',(5.09267659494215,-3.67194351384352,3.16483831483556));
#18313=CARTESIAN_POINT('Ctrl Pts',(5.06334698391922,-4.20438701666129,3.23582633137519));
#18314=CARTESIAN_POINT('Ctrl Pts',(5.31996060248519,-4.66840757573284,3.30640065967282));
#18315=CARTESIAN_POINT('Ctrl Pts',(5.78190061537116,-4.92314894439882,3.37659959628945));
#18316=CARTESIAN_POINT('Ctrl Pts',(6.30602360446337,-4.8934194778442,3.44647512179493));
#18317=CARTESIAN_POINT('Ctrl Pts',(6.73235320697049,-4.59059886848916,3.51606957003369));
#18318=CARTESIAN_POINT('Ctrl Pts',(6.93158527369931,-4.10903724627938,3.58543222201393));
#18319=CARTESIAN_POINT('Ctrl Pts',(6.84437087172348,-3.5966316690937,3.65461147199652));
#18320=CARTESIAN_POINT('Ctrl Pts',(6.4986005712581,-3.20987659405636,3.72365772216215));
#18321=CARTESIAN_POINT('Ctrl Pts',(6.00069620889802,-3.06649917569834,3.79262193940454));
#18322=CARTESIAN_POINT('Ctrl Pts',(5.50298206081782,-3.20985050236122,3.86155519007754));
#18323=CARTESIAN_POINT('Ctrl Pts',(5.17058746032825,-3.58189591316552,3.9279559301895));
#18324=CARTESIAN_POINT('Ctrl Pts',(5.09161084911067,-3.97403244462459,3.98163982698735));
#18325=CARTESIAN_POINT('Ctrl Pts',(5.13710290917312,-4.23088993114173,4.01747369242388));
#18326=CARTESIAN_POINT('Ctrl Pts',(5.18955604905821,-4.36957304831134,4.03796514432227));
#18327=CARTESIAN_POINT('Ctrl Pts',(5.29342590228157,-4.56638378889049,4.06871725914488));
#18328=CARTESIAN_POINT('Ctrl Pts',(5.53958614449405,-4.80683581259022,4.11489405980733));
#18329=CARTESIAN_POINT('Ctrl Pts',(5.98240799870313,-4.93159290708471,4.17664221174671));
#18330=CARTESIAN_POINT('Ctrl Pts',(6.43251496390311,-4.82915258042553,4.23858449276294));
#18331=CARTESIAN_POINT('Ctrl Pts',(6.75076512217874,-4.54803787118636,4.29557302280714));
#18332=CARTESIAN_POINT('Ctrl Pts',(6.90350439608594,-4.1976580738955,4.34757883005092));
#18333=CARTESIAN_POINT('Ctrl Pts',(6.91672786492714,-3.85270518195888,4.39454228245137));
#18334=CARTESIAN_POINT('Ctrl Pts',(6.80221870211402,-3.52577730207959,4.44168103975221));
#18335=CARTESIAN_POINT('Ctrl Pts',(6.55050308426461,-3.23240263631744,4.4942637068826));
#18336=CARTESIAN_POINT('Ctrl Pts',(6.1559407673884,-3.05405612320139,4.55238887331135));
#18337=CARTESIAN_POINT('Ctrl Pts',(5.68186673349783,-3.08924643489957,4.61617826163733));
#18338=CARTESIAN_POINT('Ctrl Pts',(5.36384514849828,-3.29450208863786,4.66698585997441));
#18339=CARTESIAN_POINT('Ctrl Pts',(5.19788403496136,-3.51112297261418,4.704601695143));
#18340=CARTESIAN_POINT('Ctrl Pts',(5.09206016360501,-3.72033550049983,4.73692459134345));
#18341=CARTESIAN_POINT('Ctrl Pts',(5.03646402164839,-4.01321713560672,4.77748324312575));
#18342=CARTESIAN_POINT('Ctrl Pts',(5.10326084825423,-4.36654385903782,4.82640948098865));
#18343=CARTESIAN_POINT('Ctrl Pts',(5.29537719841234,-4.67285861362723,4.87559956298535));
#18344=CARTESIAN_POINT('Ctrl Pts',(5.58777289090629,-4.88870901734329,4.92506008683499));
#18345=CARTESIAN_POINT('Ctrl Pts',(5.94094293939234,-4.98377199421309,4.97479853966587));
#18346=CARTESIAN_POINT('Ctrl Pts',(6.30598645054714,-4.94246709481662,5.0248192914387));
#18347=CARTESIAN_POINT('Ctrl Pts',(6.74299909696092,-4.71334423715881,5.0918971423708));
#18348=CARTESIAN_POINT('Ctrl Pts',(7.07217428481599,-4.14811709402513,5.17646845460267));
#18349=CARTESIAN_POINT('Ctrl Pts',(6.89663854890958,-3.37095216653505,5.27914241536394));
#18350=CARTESIAN_POINT('Ctrl Pts',(6.34353600825991,-2.99345577262945,5.36570002215199));
#18351=CARTESIAN_POINT('Ctrl Pts',(5.83000485848951,-2.97563765967302,5.43554273377057));
#18352=CARTESIAN_POINT('Ctrl Pts',(5.42395250164482,-3.11665383947864,5.49407446014151));
#18353=CARTESIAN_POINT('Ctrl Pts',(5.07781352815922,-3.45348334377841,5.55887851989237));
#18354=CARTESIAN_POINT('Ctrl Pts',(4.92119569589212,-3.96053443240852,5.63008962860051));
#18355=CARTESIAN_POINT('Ctrl Pts',(5.00900201580092,-4.39683944226663,5.68985207204882));
#18356=CARTESIAN_POINT('Ctrl Pts',(5.17540309970581,-4.65387162944169,5.7319018911364));
#18357=CARTESIAN_POINT('Ctrl Pts',(5.29550761861826,-4.78012386768163,5.75599031365937));
#18358=CARTESIAN_POINT('Ctrl Pts',(5.49807304938454,-4.94616553552845,5.79218348973528));
#18359=CARTESIAN_POINT('Ctrl Pts',(5.87591495189871,-5.09483660418974,5.84669780842769));
#18360=CARTESIAN_POINT('Ctrl Pts',(6.37161693207542,-5.03311956022957,5.91374966034583));
#18361=CARTESIAN_POINT('Ctrl Pts',(6.75295541512623,-4.79334050443991,5.97502993095026));
#18362=CARTESIAN_POINT('Ctrl Pts',(6.9948086761482,-4.46601711692582,6.03041678164421));
#18363=CARTESIAN_POINT('Ctrl Pts',(7.10079809559249,-4.07117534641981,6.08603676959893));
#18364=CARTESIAN_POINT('Ctrl Pts',(7.0550052284071,-3.66335712376636,6.14187488824605));
#18365=CARTESIAN_POINT('Ctrl Pts',(6.86254272821113,-3.29919610730441,6.19792289616172));
#18366=CARTESIAN_POINT('Ctrl Pts',(6.54938376947623,-3.02931907732678,6.25416911836834));
#18367=CARTESIAN_POINT('Ctrl Pts',(6.1579486558425,-2.89248546959741,6.31060244716706));
#18368=CARTESIAN_POINT('Ctrl Pts',(5.67285796098016,-2.91005237096891,6.37664094306513));
#18369=CARTESIAN_POINT('Ctrl Pts',(5.17447535525086,-3.18410669330449,6.4523908315935));
#18370=CARTESIAN_POINT('Ctrl Pts',(4.86359518381245,-3.74699626482779,6.53792551889047));
#18371=CARTESIAN_POINT('Ctrl Pts',(4.89358978229736,-4.28284509764931,6.60942647452156));
#18372=CARTESIAN_POINT('Ctrl Pts',(5.08616754915788,-4.65413963922357,6.66674144768274));
#18373=CARTESIAN_POINT('Ctrl Pts',(5.32539997681471,-4.90762443384318,6.71455792748918));
#18374=CARTESIAN_POINT('Ctrl Pts',(5.66770904279484,-5.08864325266815,6.76722197047057));
#18375=CARTESIAN_POINT('Ctrl Pts',(6.08751475108002,-5.13588298949551,6.82473049674227));
#18376=CARTESIAN_POINT('Ctrl Pts',(6.5645861835624,-5.00869269277779,6.891883208414));
#18377=CARTESIAN_POINT('Ctrl Pts',(6.99480434755378,-4.62476574907813,6.96867942951375));
#18378=CARTESIAN_POINT('Ctrl Pts',(7.17439385392664,-4.000445623383,7.05510766898402));
#18379=CARTESIAN_POINT('Ctrl Pts',(6.99478104501133,-3.37709835463719,7.14150114377049));
#18380=CARTESIAN_POINT('Ctrl Pts',(6.51124152718936,-2.94487966771886,7.2278171181847));
#18381=CARTESIAN_POINT('Ctrl Pts',(5.87300157020658,-2.83697217244672,7.31399284682077));
#18382=CARTESIAN_POINT('Ctrl Pts',(5.27624103646301,-3.08421455661578,7.39998347287708));
#18383=CARTESIAN_POINT('Ctrl Pts',(4.90381274036846,-3.60985955031299,7.48574172113935));
#18384=CARTESIAN_POINT('Ctrl Pts',(4.86781101481599,-4.25096067395124,7.57122146774242));
#18385=CARTESIAN_POINT('Ctrl Pts',(5.17774894918109,-4.81069654524739,7.6563808117967));
#18386=CARTESIAN_POINT('Ctrl Pts',(5.73539207552131,-5.11843269669984,7.74116666788786));
#18387=CARTESIAN_POINT('Ctrl Pts',(6.36818899742731,-5.08242658049411,7.82554016071411));
#18388=CARTESIAN_POINT('Ctrl Pts',(6.88223000977129,-4.71728080679399,7.90946350349862));
#18389=CARTESIAN_POINT('Ctrl Pts',(7.12127708571697,-4.13791637661882,7.9928932228046));
#18390=CARTESIAN_POINT('Ctrl Pts',(7.01656472861822,-3.52409769071585,8.07579754700462));
#18391=CARTESIAN_POINT('Ctrl Pts',(6.60378953069044,-3.0631252600952,8.15814989617874));
#18392=CARTESIAN_POINT('Ctrl Pts',(6.01351012908046,-2.89387326118091,8.23991854958376));
#18393=CARTESIAN_POINT('Ctrl Pts',(5.42751466531372,-3.06292659016434,8.32108499418846));
#18394=CARTESIAN_POINT('Ctrl Pts',(5.04001126571795,-3.49787745920239,8.39863860309313));
#18395=CARTESIAN_POINT('Ctrl Pts',(4.93170509712578,-4.03860077006941,8.47265039810351));
#18396=CARTESIAN_POINT('Ctrl Pts',(5.0866102730624,-4.5407113707165,8.54318119360061));
#18397=CARTESIAN_POINT('Ctrl Pts',(5.42936100250732,-4.87403779849933,8.60735376890046));
#18398=CARTESIAN_POINT('Ctrl Pts',(5.83158616216201,-5.01427171038084,8.66530592755971));
#18399=CARTESIAN_POINT('Ctrl Pts',(6.21244337123709,-4.9999360439205,8.71716546435109));
#18400=CARTESIAN_POINT('Ctrl Pts',(6.5596673206854,-4.84811610405237,8.76872530395661));
#18401=CARTESIAN_POINT('Ctrl Pts',(6.82593444340501,-4.58159404350882,8.81998719323947));
#18402=CARTESIAN_POINT('Ctrl Pts',(6.97555097229746,-4.23818719630342,8.87095217885581));
#18403=CARTESIAN_POINT('Ctrl Pts',(6.98928103115449,-3.86603752953955,8.92162246922555));
#18404=CARTESIAN_POINT('Ctrl Pts',(6.86680877161237,-3.51661440857094,8.97200097582266));
#18405=CARTESIAN_POINT('Ctrl Pts',(6.62652276655028,-3.23769642671214,9.02209139324216));
#18406=CARTESIAN_POINT('Ctrl Pts',(6.30278853986408,-3.066814257131,9.07189819214372));
#18407=CARTESIAN_POINT('Ctrl Pts',(5.94102919446653,-3.02624740788871,9.12142652419554));
#18408=CARTESIAN_POINT('Ctrl Pts',(5.59139099220371,-3.12012203285758,9.17068242089275));
#18409=CARTESIAN_POINT('Ctrl Pts',(5.30176852740219,-3.33409677722697,9.21967228892019));
#18410=CARTESIAN_POINT('Ctrl Pts',(5.11137229937622,-3.6374484355137,9.26840399241005));
#18411=CARTESIAN_POINT('Ctrl Pts',(5.04522577317681,-3.98765556961418,9.31688436084706));
#18412=CARTESIAN_POINT('Ctrl Pts',(5.11140993276018,-4.3359118298156,9.36512475134174));
#18413=CARTESIAN_POINT('Ctrl Pts',(5.32001499181377,-4.66799152448505,9.41846713475402));
#18414=CARTESIAN_POINT('Ctrl Pts',(5.68522837066175,-4.90377380153277,9.47682628398783));
#18415=CARTESIAN_POINT('Ctrl Pts',(6.15572665009444,-4.93842778603278,9.54011788753042));
#18416=CARTESIAN_POINT('Ctrl Pts',(6.48054112448135,-4.79164030355885,9.58798704654535));
#18417=CARTESIAN_POINT('Ctrl Pts',(6.65464130933801,-4.63128846987969,9.62066963734384));
#18418=CARTESIAN_POINT('Ctrl Pts',(6.76252419033915,-4.49981139232218,9.64416932945342));
#18419=CARTESIAN_POINT('Ctrl Pts',(6.90041745117454,-4.23395162044738,9.68520793907203));
#18420=CARTESIAN_POINT('Ctrl Pts',(6.92488338590534,-3.79600782000729,9.7436137313988));
#18421=CARTESIAN_POINT('Ctrl Pts',(6.67096107275452,-3.33726536059452,9.81338971644578));
#18422=CARTESIAN_POINT('Ctrl Pts',(6.2137581090805,-3.08487281006037,9.88290182303105));
#18423=CARTESIAN_POINT('Ctrl Pts',(5.69400607020532,-3.11435421989238,9.95220006390264));
#18424=CARTESIAN_POINT('Ctrl Pts',(5.27034711588601,-3.41482578093218,10.0213303098789));
#18425=CARTESIAN_POINT('Ctrl Pts',(5.0720867380328,-3.89402097251012,10.0903392614919));
#18426=CARTESIAN_POINT('Ctrl Pts',(5.15887741676057,-4.40470662845712,10.1592876980663));
#18427=CARTESIAN_POINT('Ctrl Pts',(5.50401868453627,-4.79094481054898,10.228222582476));
#18428=CARTESIAN_POINT('Ctrl Pts',(6.00198308450928,-4.93447537956818,10.297197459271));
#18429=CARTESIAN_POINT('Ctrl Pts',(6.50066246085064,-4.79094442895005,10.3662628212364));
#18430=CARTESIAN_POINT('Ctrl Pts',(6.8472808539946,-4.4033400083843,10.4354699282555));
#18431=CARTESIAN_POINT('Ctrl Pts',(6.93484780248239,-3.88932387200705,10.5048686867946));
#18432=CARTESIAN_POINT('Ctrl Pts',(6.73486307134074,-3.40581622442059,10.5745079681309));
#18433=CARTESIAN_POINT('Ctrl Pts',(6.30656413212906,-3.10151906733419,10.6444355131787));
#18434=CARTESIAN_POINT('Ctrl Pts',(5.77947299474872,-3.07154831166864,10.714696453497));
#18435=CARTESIAN_POINT('Ctrl Pts',(5.31478999974729,-3.32791188545808,10.785335947611));
#18436=CARTESIAN_POINT('Ctrl Pts',(5.05597365417069,-3.79497493605006,10.8563922532882));
#18437=CARTESIAN_POINT('Ctrl Pts',(5.08587069642077,-4.3314820844115,10.9279113545464));
#18438=CARTESIAN_POINT('Ctrl Pts',(5.39837456971601,-4.77309564174969,10.9999287051914));
#18439=CARTESIAN_POINT('Ctrl Pts',(5.90171757367533,-4.98215829124314,11.0724701515572));
#18440=CARTESIAN_POINT('Ctrl Pts',(6.4432028732693,-4.89091322567894,11.1455775949948));
#18441=CARTESIAN_POINT('Ctrl Pts',(6.85641784710808,-4.52222909517366,11.2192551426726));
#18442=CARTESIAN_POINT('Ctrl Pts',(6.95974791691079,-4.16531628624991,11.2688068655971));
#18443=CARTESIAN_POINT('Ctrl Pts',(6.95977214909355,-3.98531368433122,11.2936565383859));
#18444=CARTESIAN_POINT('Ctrl Pts',(7.04959557699666,-4.01407739529388,2.80202024039622));
#18445=CARTESIAN_POINT('Ctrl Pts',(7.04956913822907,-3.81768336112141,2.82913277892384));
#18446=CARTESIAN_POINT('Ctrl Pts',(6.9367202622634,-3.42769410118136,2.88327931957377));
#18447=CARTESIAN_POINT('Ctrl Pts',(6.48516094749322,-3.0248175347279,2.96379344062057));
#18448=CARTESIAN_POINT('Ctrl Pts',(5.89336937954221,-2.92510533993989,3.04369509984053));
#18449=CARTESIAN_POINT('Ctrl Pts',(5.34372152306085,-3.15350875728527,3.12292785038527));
#18450=CARTESIAN_POINT('Ctrl Pts',(5.00270118788897,-3.63538461147314,3.20150168364572));
#18451=CARTESIAN_POINT('Ctrl Pts',(4.9707269774799,-4.2196676866048,3.2794028151618));
#18452=CARTESIAN_POINT('Ctrl Pts',(5.25175807656894,-4.72729550009722,3.35663469084281));
#18453=CARTESIAN_POINT('Ctrl Pts',(5.75566327080534,-5.00482201266583,3.43319899049717));
#18454=CARTESIAN_POINT('Ctrl Pts',(6.32490283312075,-4.97217868326178,3.50910125356791));
#18455=CARTESIAN_POINT('Ctrl Pts',(6.78559126572007,-4.64446921311548,3.58435264375379));
#18456=CARTESIAN_POINT('Ctrl Pts',(6.99947417356179,-4.12635582910261,3.65896738189));
#18457=CARTESIAN_POINT('Ctrl Pts',(6.90573630851746,-3.57844037550777,3.73296376784759));
#18458=CARTESIAN_POINT('Ctrl Pts',(6.53785050039439,-3.16771161668764,3.80636369579688));
#18459=CARTESIAN_POINT('Ctrl Pts',(6.01199576895297,-3.01684493282177,3.87919245676609));
#18460=CARTESIAN_POINT('Ctrl Pts',(5.49033214833547,-3.16768487910272,3.95147922807082));
#18461=CARTESIAN_POINT('Ctrl Pts',(5.14483056253905,-3.55524231144764,4.02059698653933));
#18462=CARTESIAN_POINT('Ctrl Pts',(5.0635938893428,-3.96044031254016,4.07607444285223));
#18463=CARTESIAN_POINT('Ctrl Pts',(5.1104030580457,-4.22437750124471,4.11290332834221));
#18464=CARTESIAN_POINT('Ctrl Pts',(5.16416796568317,-4.36650518820908,4.13390550744089));
#18465=CARTESIAN_POINT('Ctrl Pts',(5.27044638425171,-4.56784578375605,4.16536782181109));
#18466=CARTESIAN_POINT('Ctrl Pts',(5.52142748309971,-4.81253448522336,4.21242232862903));
#18467=CARTESIAN_POINT('Ctrl Pts',(5.96924076086895,-4.9382410071469,4.27485485012556));
#18468=CARTESIAN_POINT('Ctrl Pts',(6.42087513852533,-4.83500709645662,4.3370303440752));
#18469=CARTESIAN_POINT('Ctrl Pts',(6.73765110446275,-4.55466041922396,4.39381972192088));
#18470=CARTESIAN_POINT('Ctrl Pts',(6.88864417341743,-4.20781172341044,4.44529669035746));
#18471=CARTESIAN_POINT('Ctrl Pts',(6.90147923264546,-3.86824513057332,4.49153432087195));
#18472=CARTESIAN_POINT('Ctrl Pts',(6.78923182972319,-3.54825327547411,4.53768901187963));
#18473=CARTESIAN_POINT('Ctrl Pts',(6.54396727764667,-3.26270069623157,4.58889957043465));
#18474=CARTESIAN_POINT('Ctrl Pts',(6.16200255235145,-3.09043995215812,4.64515540035398));
#18475=CARTESIAN_POINT('Ctrl Pts',(5.70640445778069,-3.12464870133968,4.70646763990055));
#18476=CARTESIAN_POINT('Ctrl Pts',(5.40286749556076,-3.32088745545974,4.75500864335017));
#18477=CARTESIAN_POINT('Ctrl Pts',(5.24512838139169,-3.5268208069634,4.79077034626969));
#18478=CARTESIAN_POINT('Ctrl Pts',(5.14477881719594,-3.72525665024375,4.82142974515389));
#18479=CARTESIAN_POINT('Ctrl Pts',(5.09234818824701,-4.00210562688859,4.85977002075827));
#18480=CARTESIAN_POINT('Ctrl Pts',(5.15533182225625,-4.33458130178686,4.90581914691398));
#18481=CARTESIAN_POINT('Ctrl Pts',(5.33548776796468,-4.6215748362361,4.95192433144584));
#18482=CARTESIAN_POINT('Ctrl Pts',(5.60848260587076,-4.82296944796147,4.99809986716363));
#18483=CARTESIAN_POINT('Ctrl Pts',(5.9369440104669,-4.91125654772996,5.04435881769998));
#18484=CARTESIAN_POINT('Ctrl Pts',(6.27520360585225,-4.87289052404234,5.0907169889183));
#18485=CARTESIAN_POINT('Ctrl Pts',(6.6787996200642,-4.66111658918346,5.15267727991992));
#18486=CARTESIAN_POINT('Ctrl Pts',(6.98098150122638,-4.14106395747072,5.23045754094985));
#18487=CARTESIAN_POINT('Ctrl Pts',(6.81977626230843,-3.43017766460645,5.32440599363029));
#18488=CARTESIAN_POINT('Ctrl Pts',(6.31552816547733,-3.08645665568759,5.40330039236375));
#18489=CARTESIAN_POINT('Ctrl Pts',(5.84855411100682,-3.07029855427464,5.46681774835805));
#18490=CARTESIAN_POINT('Ctrl Pts',(5.4797268769858,-3.19842337273609,5.51998686657359));
#18491=CARTESIAN_POINT('Ctrl Pts',(5.16567222350704,-3.50409863861733,5.57879374554913));
#18492=CARTESIAN_POINT('Ctrl Pts',(5.02366796970531,-3.96389006248025,5.64337126252039));
#18493=CARTESIAN_POINT('Ctrl Pts',(5.1032679493576,-4.35943860083833,5.69755174644111));
#18494=CARTESIAN_POINT('Ctrl Pts',(5.25414338424139,-4.59250987985455,5.7356818133743));
#18495=CARTESIAN_POINT('Ctrl Pts',(5.3630668329631,-4.70701089826391,5.75752797728752));
#18496=CARTESIAN_POINT('Ctrl Pts',(5.54680053310836,-4.85761941833764,5.79035698196648));
#18497=CARTESIAN_POINT('Ctrl Pts',(5.88965278851035,-4.9925747646598,5.83982581730757));
#18498=CARTESIAN_POINT('Ctrl Pts',(6.33999449822917,-4.93659055838853,5.90073991716705));
#18499=CARTESIAN_POINT('Ctrl Pts',(6.6869391381759,-4.71851451977266,5.95648601990599));
#18500=CARTESIAN_POINT('Ctrl Pts',(6.90731245937833,-4.42035144578017,6.00694356452062));
#18501=CARTESIAN_POINT('Ctrl Pts',(7.00409117035043,-4.06008469798609,6.05769403505103));
#18502=CARTESIAN_POINT('Ctrl Pts',(6.96230174690874,-3.68725672811026,6.10873851183451));
#18503=CARTESIAN_POINT('Ctrl Pts',(6.78606403741209,-3.35362517017195,6.16007991043999));
#18504=CARTESIAN_POINT('Ctrl Pts',(6.49860389913839,-3.10577421388223,6.21171855444694));
#18505=CARTESIAN_POINT('Ctrl Pts',(6.13835846199652,-2.97974364176408,6.26365546641588));
#18506=CARTESIAN_POINT('Ctrl Pts',(5.69070282319273,-2.99583565516249,6.32459628110795));
#18507=CARTESIAN_POINT('Ctrl Pts',(5.22903186486354,-3.24932298263957,6.39473487294707));
#18508=CARTESIAN_POINT('Ctrl Pts',(4.93943407798838,-3.77280013860123,6.47430161545231));
#18509=CARTESIAN_POINT('Ctrl Pts',(4.96712454271302,-4.27383503035714,6.54114965025572));
#18510=CARTESIAN_POINT('Ctrl Pts',(5.14782487662629,-4.62241497626213,6.59494409855566));
#18511=CARTESIAN_POINT('Ctrl Pts',(5.37295079462874,-4.86103853161568,6.63994694552246));
#18512=CARTESIAN_POINT('Ctrl Pts',(5.69611194962567,-5.03208597410825,6.68966723228357));
#18513=CARTESIAN_POINT('Ctrl Pts',(6.09404105102488,-5.07700452575227,6.74417783171338));
#18514=CARTESIAN_POINT('Ctrl Pts',(6.54806597605186,-4.95615077255924,6.80807397654506));
#18515=CARTESIAN_POINT('Ctrl Pts',(6.95984908440191,-4.58929774796911,6.88152070079881));
#18516=CARTESIAN_POINT('Ctrl Pts',(7.13324602081489,-3.98862814197939,6.96467721107475));
#18517=CARTESIAN_POINT('Ctrl Pts',(6.9598216073969,-3.38470802488132,7.04834227232992));
#18518=CARTESIAN_POINT('Ctrl Pts',(6.48881513689751,-2.96289006313062,7.13247292529825));
#18519=CARTESIAN_POINT('Ctrl Pts',(5.86248371502993,-2.85639547254553,7.21704160193825));
#18520=CARTESIAN_POINT('Ctrl Pts',(5.27257813080996,-3.10013645753721,7.30200242561844));
#18521=CARTESIAN_POINT('Ctrl Pts',(4.90156434344046,-3.62273164012634,7.38731106651996));
#18522=CARTESIAN_POINT('Ctrl Pts',(4.86488076919295,-4.26484215361151,7.47291989869636));
#18523=CARTESIAN_POINT('Ctrl Pts',(5.17689565992446,-4.82960611614006,7.55877747642911));
#18524=CARTESIAN_POINT('Ctrl Pts',(5.74278059709062,-5.14259803736158,7.64484502388108));
#18525=CARTESIAN_POINT('Ctrl Pts',(6.38962394316408,-5.1063947491349,7.73106975793031));
#18526=CARTESIAN_POINT('Ctrl Pts',(6.91886767714568,-4.73119514243953,7.81739789224607));
#18527=CARTESIAN_POINT('Ctrl Pts',(7.16697506945629,-4.13139347086528,7.90378793880489));
#18528=CARTESIAN_POINT('Ctrl Pts',(7.05840291902035,-3.49156698921832,7.99018524187825));
#18529=CARTESIAN_POINT('Ctrl Pts',(6.6259671749691,-3.00779841905544,8.07653128299141));
#18530=CARTESIAN_POINT('Ctrl Pts',(6.00342339258711,-2.82875695864265,8.16278221624947));
#18531=CARTESIAN_POINT('Ctrl Pts',(5.3816245849515,-3.00760289250318,8.24887562077341));
#18532=CARTESIAN_POINT('Ctrl Pts',(4.96793364487745,-3.47126919190322,8.33159562484918));
#18533=CARTESIAN_POINT('Ctrl Pts',(4.85154007935987,-4.05076879557578,8.41090797936888));
#18534=CARTESIAN_POINT('Ctrl Pts',(5.01800897195225,-4.59134836316443,8.48682542635688));
#18535=CARTESIAN_POINT('Ctrl Pts',(5.38828999036735,-4.95178056335741,8.55617651731747));
#18536=CARTESIAN_POINT('Ctrl Pts',(5.82439623786284,-5.10394949210358,8.61901205223471));
#18537=CARTESIAN_POINT('Ctrl Pts',(6.23842569304392,-5.08845315445427,8.6753812452482));
#18538=CARTESIAN_POINT('Ctrl Pts',(6.61685601287741,-4.92308289439992,8.73156765404928));
#18539=CARTESIAN_POINT('Ctrl Pts',(6.90771592127364,-4.63205020805392,8.78754987472152));
#18540=CARTESIAN_POINT('Ctrl Pts',(7.07151318879937,-4.2562632267042,8.84332122014839));
#18541=CARTESIAN_POINT('Ctrl Pts',(7.08662361123704,-3.84826122336414,8.89887039673394));
#18542=CARTESIAN_POINT('Ctrl Pts',(6.95218526115907,-3.46454996619298,8.95418779366907));
#18543=CARTESIAN_POINT('Ctrl Pts',(6.68800360958442,-3.15783352136326,9.00926396892089));
#18544=CARTESIAN_POINT('Ctrl Pts',(6.33164898032002,-2.96969809280073,9.06409031981465));
#18545=CARTESIAN_POINT('Ctrl Pts',(5.93307270473151,-2.92498136414862,9.11865878717923));
#18546=CARTESIAN_POINT('Ctrl Pts',(5.54760066898876,-3.028464827269,9.17296209959429));
#18547=CARTESIAN_POINT('Ctrl Pts',(5.22817429689392,-3.26445713236173,9.22699350570149));
#18548=CARTESIAN_POINT('Ctrl Pts',(5.01816505797095,-3.59907103783072,9.28074733097771));
#18549=CARTESIAN_POINT('Ctrl Pts',(4.94523109104339,-3.98531889354533,9.33421783283799));
#18550=CARTESIAN_POINT('Ctrl Pts',(5.01822063845842,-4.36924877748871,9.3874017867631));
#18551=CARTESIAN_POINT('Ctrl Pts',(5.24807831595622,-4.73508877868424,9.44617162792128));
#18552=CARTESIAN_POINT('Ctrl Pts',(5.65005396981199,-4.99449121289196,9.51039938577164));
#18553=CARTESIAN_POINT('Ctrl Pts',(6.16696735742553,-5.03242068584373,9.57993815379645));
#18554=CARTESIAN_POINT('Ctrl Pts',(6.52296885884133,-4.87140435012961,9.63241396136568));
#18555=CARTESIAN_POINT('Ctrl Pts',(6.71347179503556,-4.69592899910923,9.66817929864774));
#18556=CARTESIAN_POINT('Ctrl Pts',(6.83142515980489,-4.55217041674898,9.69387451281195));
#18557=CARTESIAN_POINT('Ctrl Pts',(6.98197740508559,-4.26180022510805,9.7386956488303));
#18558=CARTESIAN_POINT('Ctrl Pts',(7.00835664843526,-3.78482966702737,9.80230908785757));
#18559=CARTESIAN_POINT('Ctrl Pts',(6.73265925800214,-3.28750526053974,9.87798665633685));
#18560=CARTESIAN_POINT('Ctrl Pts',(6.23900967174894,-3.01545842822921,9.9530177739628));
#18561=CARTESIAN_POINT('Ctrl Pts',(5.68107426992735,-3.04754329136254,10.02741686381));
#18562=CARTESIAN_POINT('Ctrl Pts',(5.22919452226571,-3.36862150726833,10.1012057629823));
#18563=CARTESIAN_POINT('Ctrl Pts',(5.01940446719196,-3.87702307203514,10.1744097575186));
#18564=CARTESIAN_POINT('Ctrl Pts',(5.11135737798824,-4.41486364909888,10.2470495853014));
#18565=CARTESIAN_POINT('Ctrl Pts',(5.47273125967169,-4.81842416402667,10.3191579186434));
#18566=CARTESIAN_POINT('Ctrl Pts',(5.98976976867957,-4.96684498725752,10.3907666330935));
#18567=CARTESIAN_POINT('Ctrl Pts',(6.50319689175154,-4.81844594629322,10.4619122586038));
#18568=CARTESIAN_POINT('Ctrl Pts',(6.85686854910234,-4.4220387290267,10.5326333401887));
#18569=CARTESIAN_POINT('Ctrl Pts',(6.94499280492971,-3.90107632051501,10.6029711277556));
#18570=CARTESIAN_POINT('Ctrl Pts',(6.74345059478189,-3.41542481303838,10.6729692924891));
#18571=CARTESIAN_POINT('Ctrl Pts',(6.31626083963058,-3.11267459898931,10.742672972225));
#18572=CARTESIAN_POINT('Ctrl Pts',(5.79529421647195,-3.08367324798476,10.8121304684942));
#18573=CARTESIAN_POINT('Ctrl Pts',(5.34009144913045,-3.33549309978965,10.8813884178955));
#18574=CARTESIAN_POINT('Ctrl Pts',(5.08895191849142,-3.78995661189334,10.9505018220951));
#18575=CARTESIAN_POINT('Ctrl Pts',(5.11835951367094,-4.30749747225698,11.0195109289986));
#18576=CARTESIAN_POINT('Ctrl Pts',(5.41801944296879,-4.73002031986431,11.0884703947198));
#18577=CARTESIAN_POINT('Ctrl Pts',(5.89668467049593,-4.92825270792295,11.157438280058));
#18578=CARTESIAN_POINT('Ctrl Pts',(6.40782870093169,-4.84169521275955,11.2264591709475));
#18579=CARTESIAN_POINT('Ctrl Pts',(6.79515456050063,-4.4954187626051,11.2955952685095));
#18580=CARTESIAN_POINT('Ctrl Pts',(6.89129509472742,-4.16277368800117,11.3417786308327));
#18581=CARTESIAN_POINT('Ctrl Pts',(6.89131766144517,-3.99514256899045,11.3649203988529));
#18582=CARTESIAN_POINT('Ctrl Pts',(7.11181302032296,-4.0034772816564,2.72529728340312));
#18583=CARTESIAN_POINT('Ctrl Pts',(7.11178503697032,-3.795609668472,2.75399376949983));
#18584=CARTESIAN_POINT('Ctrl Pts',(6.99231662213726,-3.38176503061251,2.8114460028125));
#18585=CARTESIAN_POINT('Ctrl Pts',(6.51087276301266,-2.95155110950397,2.89735412612978));
#18586=CARTESIAN_POINT('Ctrl Pts',(5.87632413377557,-2.84418543881411,2.98303979398471));
#18587=CARTESIAN_POINT('Ctrl Pts',(5.2839166060325,-3.08988019972769,3.06841725271835));
#18588=CARTESIAN_POINT('Ctrl Pts',(4.91451380684877,-3.61116286149957,3.15345799266807));
#18589=CARTESIAN_POINT('Ctrl Pts',(4.87941312230243,-4.24603397475997,3.23810978758372));
#18590=CARTESIAN_POINT('Ctrl Pts',(5.18560875700521,-4.79977729807461,3.3223375500771));
#18591=CARTESIAN_POINT('Ctrl Pts',(5.73675144209106,-5.10364461823107,3.4061038382733));
#18592=CARTESIAN_POINT('Ctrl Pts',(6.36119748488511,-5.06806408189714,3.48936636705102));
#18593=CARTESIAN_POINT('Ctrl Pts',(6.86777018966466,-4.70793950062804,3.57209524538133));
#18594=CARTESIAN_POINT('Ctrl Pts',(7.10342410685789,-4.13743665807794,3.65425938248879));
#18595=CARTESIAN_POINT('Ctrl Pts',(7.00016590193463,-3.53336934983432,3.73583291487668));
#18596=CARTESIAN_POINT('Ctrl Pts',(6.59438611967027,-3.08027854269764,3.81679253233116));
#18597=CARTESIAN_POINT('Ctrl Pts',(6.01433584924907,-2.91387555126545,3.89711903146131));
#18598=CARTESIAN_POINT('Ctrl Pts',(5.43928254017653,-3.08021570651043,3.97679647255008));
#18599=CARTESIAN_POINT('Ctrl Pts',(5.05895974480875,-3.5069990781973,4.0528868562602));
#18600=CARTESIAN_POINT('Ctrl Pts',(4.96976763296824,-3.95237190959014,4.11385288434471));
#18601=CARTESIAN_POINT('Ctrl Pts',(5.0211552143318,-4.24201596307504,4.15426621773676));
#18602=CARTESIAN_POINT('Ctrl Pts',(5.08010879807319,-4.39785530700753,4.17729369334087));
#18603=CARTESIAN_POINT('Ctrl Pts',(5.19657114195399,-4.6184869703178,4.21176842639279));
#18604=CARTESIAN_POINT('Ctrl Pts',(5.47119125599088,-4.88607017711824,4.26322384295608));
#18605=CARTESIAN_POINT('Ctrl Pts',(5.95966222257167,-5.02298665218075,4.33131168944356));
#18606=CARTESIAN_POINT('Ctrl Pts',(6.45043526956446,-4.91056588865359,4.39887225762002));
#18607=CARTESIAN_POINT('Ctrl Pts',(6.79314941065994,-4.60696622071268,4.46032348296662));
#18608=CARTESIAN_POINT('Ctrl Pts',(6.9558334855932,-4.23292331056928,4.51582395385229));
#18609=CARTESIAN_POINT('Ctrl Pts',(6.96951025099049,-3.86809398252934,4.56548927299046));
#18610=CARTESIAN_POINT('Ctrl Pts',(6.84924354955551,-3.52565366333575,4.6148810745284));
#18611=CARTESIAN_POINT('Ctrl Pts',(6.58767150103308,-3.22134137372009,4.66946015528846));
#18612=CARTESIAN_POINT('Ctrl Pts',(6.18235541401055,-3.0388990108291,4.72912598691042));
#18613=CARTESIAN_POINT('Ctrl Pts',(5.70197393505759,-3.07534404320876,4.79377090669685));
#18614=CARTESIAN_POINT('Ctrl Pts',(5.38416977230659,-3.28116084516777,4.8445902293805));
#18615=CARTESIAN_POINT('Ctrl Pts',(5.21966595419117,-3.49597856977572,4.88188785520888));
#18616=CARTESIAN_POINT('Ctrl Pts',(5.11528011960377,-3.70245947496454,4.91378229331294));
#18617=CARTESIAN_POINT('Ctrl Pts',(5.06106882547897,-3.98943465448296,4.95351375393308));
#18618=CARTESIAN_POINT('Ctrl Pts',(5.12618530561125,-4.33220315307956,5.00098440504624));
#18619=CARTESIAN_POINT('Ctrl Pts',(5.31109273276004,-4.62645525277273,5.04825832289593));
#18620=CARTESIAN_POINT('Ctrl Pts',(5.5896728391335,-4.8317388157924,5.09534903382872));
#18621=CARTESIAN_POINT('Ctrl Pts',(5.92295480412722,-4.92113185558065,5.14227041620987));
#18622=CARTESIAN_POINT('Ctrl Pts',(6.26421131547055,-4.88225344620643,5.18903417313737));
#18623=CARTESIAN_POINT('Ctrl Pts',(6.66909695604073,-4.66950391227245,5.25119574478853));
#18624=CARTESIAN_POINT('Ctrl Pts',(6.96872410809086,-4.15143760418596,5.32855257233037));
#18625=CARTESIAN_POINT('Ctrl Pts',(6.8085865206455,-3.45225571131928,5.42097838800836));
#18626=CARTESIAN_POINT('Ctrl Pts',(6.31714251855204,-3.1186633455213,5.49774585582468));
#18627=CARTESIAN_POINT('Ctrl Pts',(5.86618303936299,-3.10330610067415,5.55908145139043));
#18628=CARTESIAN_POINT('Ctrl Pts',(5.51181006773901,-3.22658005086454,5.61016213242431));
#18629=CARTESIAN_POINT('Ctrl Pts',(5.21202969008444,-3.5188532387546,5.66633081666598));
#18630=CARTESIAN_POINT('Ctrl Pts',(5.07759303828484,-3.95538499461575,5.72761250189965));
#18631=CARTESIAN_POINT('Ctrl Pts',(5.15296720022287,-4.32855327746985,5.77872934943021));
#18632=CARTESIAN_POINT('Ctrl Pts',(5.29475280348604,-4.54747613431151,5.81454405119438));
#18633=CARTESIAN_POINT('Ctrl Pts',(5.39688304163522,-4.65482873693581,5.83502588408689));
#18634=CARTESIAN_POINT('Ctrl Pts',(5.56892779389234,-4.79583961287311,5.86576115556887));
#18635=CARTESIAN_POINT('Ctrl Pts',(5.88894832539248,-4.9215688629896,5.91191769336285));
#18636=CARTESIAN_POINT('Ctrl Pts',(6.30708827323726,-4.86933300302203,5.96847220906027));
#18637=CARTESIAN_POINT('Ctrl Pts',(6.62788735520902,-4.66753190240589,6.02001845773736));
#18638=CARTESIAN_POINT('Ctrl Pts',(6.83101003502994,-4.39254735889121,6.06654237092183));
#18639=CARTESIAN_POINT('Ctrl Pts',(6.91988771324996,-4.06130312576411,6.11319476549568));
#18640=CARTESIAN_POINT('Ctrl Pts',(6.88148404501785,-3.71943526644181,6.15999913034724));
#18641=CARTESIAN_POINT('Ctrl Pts',(6.72018765865318,-3.41426217881823,6.2069633667072));
#18642=CARTESIAN_POINT('Ctrl Pts',(6.45771684783584,-3.18804833433947,6.25410242444302));
#18643=CARTESIAN_POINT('Ctrl Pts',(6.12942429058675,-3.07326355575574,6.30142649923685));
#18644=CARTESIAN_POINT('Ctrl Pts',(5.72212261020255,-3.0879652583245,6.35687278657594));
#18645=CARTESIAN_POINT('Ctrl Pts',(5.30280188330194,-3.31834662771335,6.4205824119603));
#18646=CARTESIAN_POINT('Ctrl Pts',(5.04015910673608,-3.79329231273531,6.49276455500539));
#18647=CARTESIAN_POINT('Ctrl Pts',(5.06529254998145,-4.24752611947387,6.55336865808706));
#18648=CARTESIAN_POINT('Ctrl Pts',(5.229105522544,-4.56352145996701,6.60213508583633));
#18649=CARTESIAN_POINT('Ctrl Pts',(5.43321055638464,-4.7798606832403,6.64293592276993));
#18650=CARTESIAN_POINT('Ctrl Pts',(5.72627515597292,-4.93498617020499,6.68802792013858));
#18651=CARTESIAN_POINT('Ctrl Pts',(6.08735128746861,-4.97576489038208,6.73749113160384));
#18652=CARTESIAN_POINT('Ctrl Pts',(6.49967356053982,-4.86604225236812,6.7955213010878));
#18653=CARTESIAN_POINT('Ctrl Pts',(6.87420709747073,-4.53253993649614,6.86231193633499));
#18654=CARTESIAN_POINT('Ctrl Pts',(7.03239424791724,-3.98519320250181,6.9381046731321));
#18655=CARTESIAN_POINT('Ctrl Pts',(6.8741451200112,-3.43332696122199,7.01455824015083));
#18656=CARTESIAN_POINT('Ctrl Pts',(6.44261208450338,-3.04651151223732,7.09168325300931));
#18657=CARTESIAN_POINT('Ctrl Pts',(5.86655717868025,-2.94824980040446,7.16947724567467));
#18658=CARTESIAN_POINT('Ctrl Pts',(5.32167885280403,-3.17302008183712,7.24794249190133));
#18659=CARTESIAN_POINT('Ctrl Pts',(4.97724918654381,-3.65751078947094,7.3270742884974));
#18660=CARTESIAN_POINT('Ctrl Pts',(4.94266353869487,-4.25587662754318,7.40686673243344));
#18661=CARTESIAN_POINT('Ctrl Pts',(5.23454234061227,-4.78511199353983,7.48731081374599));
#18662=CARTESIAN_POINT('Ctrl Pts',(5.76723695574062,-5.08027341466217,7.56838248480538));
#18663=CARTESIAN_POINT('Ctrl Pts',(6.37988233163738,-5.04648348782411,7.65006374692676));
#18664=CARTESIAN_POINT('Ctrl Pts',(6.88440160593799,-4.68944269844362,7.73233497259739));
#18665=CARTESIAN_POINT('Ctrl Pts',(7.12272965880694,-4.11471198609239,7.81515815314353));
#18666=CARTESIAN_POINT('Ctrl Pts',(7.01854737810762,-3.49745445431086,7.89850602421412));
#18667=CARTESIAN_POINT('Ctrl Pts',(6.59913665512866,-3.02739537215762,7.98235325668356));
#18668=CARTESIAN_POINT('Ctrl Pts',(5.99089552939524,-2.85185547830102,8.0666537355345));
#18669=CARTESIAN_POINT('Ctrl Pts',(5.37895087333546,-3.02724577484401,8.15138435106854));
#18670=CARTESIAN_POINT('Ctrl Pts',(4.96873838061378,-3.4861291063974,8.23332981304256));
#18671=CARTESIAN_POINT('Ctrl Pts',(4.85223629310714,-4.06382045547982,8.31242873092161));
#18672=CARTESIAN_POINT('Ctrl Pts',(5.01879225277718,-4.60612524072465,8.38858506420336));
#18673=CARTESIAN_POINT('Ctrl Pts',(5.39215287487895,-4.9701201364919,8.45857688050792));
#18674=CARTESIAN_POINT('Ctrl Pts',(5.83447254628042,-5.12466841834738,8.52232192406592));
#18675=CARTESIAN_POINT('Ctrl Pts',(6.25638035377061,-5.1090579638618,8.57978038495634));
#18676=CARTESIAN_POINT('Ctrl Pts',(6.64376737701431,-4.93997081523902,8.63729012374795));
#18677=CARTESIAN_POINT('Ctrl Pts',(6.94290952660399,-4.6409000426499,8.69485452773811));
#18678=CARTESIAN_POINT('Ctrl Pts',(7.11219528325435,-4.25296279440545,8.75244998619474));
#18679=CARTESIAN_POINT('Ctrl Pts',(7.12803866414581,-3.82988735801254,8.8100627820474));
#18680=CARTESIAN_POINT('Ctrl Pts',(6.98820455924593,-3.43025618594452,8.86767703449591));
#18681=CARTESIAN_POINT('Ctrl Pts',(6.71208792131979,-3.10942500354523,8.92527773350626));
#18682=CARTESIAN_POINT('Ctrl Pts',(6.33802625218942,-2.91175521399945,8.98284944887227));
#18683=CARTESIAN_POINT('Ctrl Pts',(5.91791836782838,-2.86446190085055,9.04037715807962));
#18684=CARTESIAN_POINT('Ctrl Pts',(5.50999816880691,-2.97381056092891,9.09784552911978));
#18685=CARTESIAN_POINT('Ctrl Pts',(5.1706475163805,-3.22433555582723,9.1552402121433));
#18686=CARTESIAN_POINT('Ctrl Pts',(4.94666850851543,-3.58093351744638,9.21254527965908));
#18687=CARTESIAN_POINT('Ctrl Pts',(4.86851194638551,-3.9940613147631,9.2697490146684));
#18688=CARTESIAN_POINT('Ctrl Pts',(4.94671706804593,-4.40612531487305,9.32683105079786));
#18689=CARTESIAN_POINT('Ctrl Pts',(5.19406373867607,-4.80007560428671,9.39010930326567));
#18690=CARTESIAN_POINT('Ctrl Pts',(5.62823706810774,-5.08055728128927,9.45950840910193));
#18691=CARTESIAN_POINT('Ctrl Pts',(6.18883171995305,-5.12196510699354,9.53493153509677));
#18692=CARTESIAN_POINT('Ctrl Pts',(6.57630879888758,-4.94690033774589,9.59203839047609));
#18693=CARTESIAN_POINT('Ctrl Pts',(6.78403797218043,-4.75557641911101,9.63103661249943));
#18694=CARTESIAN_POINT('Ctrl Pts',(6.91276029943424,-4.59870147295395,9.65907726902172));
#18695=CARTESIAN_POINT('Ctrl Pts',(7.07729956347344,-4.28147376753379,9.70805109539169));
#18696=CARTESIAN_POINT('Ctrl Pts',(7.10639635228469,-3.75916764163223,9.77771384283918));
#18697=CARTESIAN_POINT('Ctrl Pts',(6.80391089471105,-3.21307570521622,9.86079704272353));
#18698=CARTESIAN_POINT('Ctrl Pts',(6.2609409806921,-2.91366124263847,9.94333528846695));
#18699=CARTESIAN_POINT('Ctrl Pts',(5.64625305798367,-2.94889736194364,10.0253000041248));
#18700=CARTESIAN_POINT('Ctrl Pts',(5.14790701284458,-3.30290571674617,10.1066660051286));
#18701=CARTESIAN_POINT('Ctrl Pts',(4.91646375369252,-3.86373001111236,10.1874119824758));
#18702=CARTESIAN_POINT('Ctrl Pts',(5.01790999463095,-4.45690610328577,10.2675187444275));
#18703=CARTESIAN_POINT('Ctrl Pts',(5.4162045723001,-4.90156974945713,10.3469724146488));
#18704=CARTESIAN_POINT('Ctrl Pts',(5.98520329484128,-5.0647656683169,10.4257622661485));
#18705=CARTESIAN_POINT('Ctrl Pts',(6.54898949352491,-4.90161790412091,10.5038818275361));
#18706=CARTESIAN_POINT('Ctrl Pts',(6.93618330712169,-4.4672853226491,10.5813283621489));
#18707=CARTESIAN_POINT('Ctrl Pts',(7.0321116791204,-3.89849452357714,10.6581033369473));
#18708=CARTESIAN_POINT('Ctrl Pts',(6.81262813853771,-3.37046494817674,10.7342117384801));
#18709=CARTESIAN_POINT('Ctrl Pts',(6.34989485304325,-3.04297798221524,10.8096633648087));
#18710=CARTESIAN_POINT('Ctrl Pts',(5.78863332577001,-3.01213943792801,10.8844698528756));
#18711=CARTESIAN_POINT('Ctrl Pts',(5.30116720621585,-3.28231261460185,10.958651011249));
#18712=CARTESIAN_POINT('Ctrl Pts',(5.03414065496795,-3.76648217455745,11.0322203362354));
#18713=CARTESIAN_POINT('Ctrl Pts',(5.0657612686785,-4.31399257613907,11.1052167694189));
#18714=CARTESIAN_POINT('Ctrl Pts',(5.38103274839073,-4.75764250667029,11.1776583648672));
#18715=CARTESIAN_POINT('Ctrl Pts',(5.88048241165544,-4.96386839430271,11.2495801905597));
#18716=CARTESIAN_POINT('Ctrl Pts',(6.40941698618055,-4.87375847765753,11.3209983713259));
#18717=CARTESIAN_POINT('Ctrl Pts',(6.80673213210873,-4.51761905992164,11.3919962517265));
#18718=CARTESIAN_POINT('Ctrl Pts',(6.90419755947852,-4.17887731899267,11.4389950778511));
#18719=CARTESIAN_POINT('Ctrl Pts',(6.90422048036531,-4.00861534543431,11.4625000399251));
#18720=CARTESIAN_POINT('Ctrl Pts',(7.08935434998871,-3.99023209767526,2.62933176205122));
#18721=CARTESIAN_POINT('Ctrl Pts',(7.08932688285949,-3.78619912616226,2.65749886918541));
#18722=CARTESIAN_POINT('Ctrl Pts',(6.97225742007367,-3.37929495075464,2.71396227449415));
#18723=CARTESIAN_POINT('Ctrl Pts',(6.4959395448978,-2.95271134548437,2.79904118774148));
#18724=CARTESIAN_POINT('Ctrl Pts',(5.86342126244207,-2.84513906790044,2.88445011210575));
#18725=CARTESIAN_POINT('Ctrl Pts',(5.26853596979891,-3.09120074560871,2.97014778749716));
#18726=CARTESIAN_POINT('Ctrl Pts',(4.89471164796743,-3.61770953674116,3.05608476471754));
#18727=CARTESIAN_POINT('Ctrl Pts',(4.85840821685399,-4.26367377675506,3.1422138288304));
#18728=CARTESIAN_POINT('Ctrl Pts',(5.17152956425176,-4.83116889517306,3.22848321087116));
#18729=CARTESIAN_POINT('Ctrl Pts',(5.73952231760977,-5.1449839685189,3.3148407995635));
#18730=CARTESIAN_POINT('Ctrl Pts',(6.38756274099376,-5.10862866433251,3.40123877203696));
#18731=CARTESIAN_POINT('Ctrl Pts',(6.91687976395631,-4.73301508245801,3.48762382685246));
#18732=CARTESIAN_POINT('Ctrl Pts',(7.16496045282747,-4.13383039277197,3.57394514348085));
#18733=CARTESIAN_POINT('Ctrl Pts',(7.05634188199328,-3.49536193020094,3.66015119897581));
#18734=CARTESIAN_POINT('Ctrl Pts',(6.62546157536257,-3.01351480304848,3.74619172902684));
#18735=CARTESIAN_POINT('Ctrl Pts',(6.00584453576659,-2.83528701623401,3.83201712057257));
#18736=CARTESIAN_POINT('Ctrl Pts',(5.38823156605757,-3.01349570186831,3.91757943615934));
#18737=CARTESIAN_POINT('Ctrl Pts',(4.9776391918564,-3.47368186406432,3.99967416531157));
#18738=CARTESIAN_POINT('Ctrl Pts',(4.88081244001865,-3.95609746742031,4.06572132496842));
#18739=CARTESIAN_POINT('Ctrl Pts',(4.93659467832656,-4.27068186833768,4.1096153344438));
#18740=CARTESIAN_POINT('Ctrl Pts',(5.00069912947771,-4.44014510684179,4.13465648931247));
#18741=CARTESIAN_POINT('Ctrl Pts',(5.12743957449684,-4.6802586444565,4.17217678554748));
#18742=CARTESIAN_POINT('Ctrl Pts',(5.42683993188746,-4.97217063644552,4.22830517648922));
#18743=CARTESIAN_POINT('Ctrl Pts',(5.96096699897456,-5.12206279818076,4.30276781882196));
#18744=CARTESIAN_POINT('Ctrl Pts',(6.49902876152345,-4.99896356644126,4.37684117025936));
#18745=CARTESIAN_POINT('Ctrl Pts',(6.87559825091274,-4.66549634791073,4.44436497611438));
#18746=CARTESIAN_POINT('Ctrl Pts',(7.05461408495889,-4.25402036572474,4.50542661030662));
#18747=CARTESIAN_POINT('Ctrl Pts',(7.06969558189068,-3.85224672374576,4.56013139070142));
#18748=CARTESIAN_POINT('Ctrl Pts',(6.93717502307927,-3.47483694654967,4.61457295672824));
#18749=CARTESIAN_POINT('Ctrl Pts',(6.64875041917917,-3.13927424785343,4.67476637000182));
#18750=CARTESIAN_POINT('Ctrl Pts',(6.20170223313162,-2.93804341964427,4.74058490002232));
#18751=CARTESIAN_POINT('Ctrl Pts',(5.67192221372407,-2.978262942237,4.81188320877822));
#18752=CARTESIAN_POINT('Ctrl Pts',(5.3215938512512,-3.2052069184109,4.86793754222562));
#18753=CARTESIAN_POINT('Ctrl Pts',(5.14042083624559,-3.44180714820557,4.90902121836561));
#18754=CARTESIAN_POINT('Ctrl Pts',(5.02550641655777,-3.66912250596354,4.94413847804827));
#18755=CARTESIAN_POINT('Ctrl Pts',(4.9659167911861,-3.98480613469966,4.98785114911865));
#18756=CARTESIAN_POINT('Ctrl Pts',(5.03749702385629,-4.36134884281863,5.04000993703854));
#18757=CARTESIAN_POINT('Ctrl Pts',(5.24037015462402,-4.68404809620616,5.09187198427612));
#18758=CARTESIAN_POINT('Ctrl Pts',(5.54537654264952,-4.90873413606796,5.14343592097922));
#18759=CARTESIAN_POINT('Ctrl Pts',(5.909472076432,-5.00629854924447,5.194701131758));
#18760=CARTESIAN_POINT('Ctrl Pts',(6.28132398727991,-4.96385799414479,5.24566981818468));
#18761=CARTESIAN_POINT('Ctrl Pts',(6.72130577810205,-4.73250966468848,5.31323388597859));
#18762=CARTESIAN_POINT('Ctrl Pts',(7.04489872138567,-4.17152523185947,5.39697306163749));
#18763=CARTESIAN_POINT('Ctrl Pts',(6.87173413710806,-3.42039959502914,5.49631993121801));
#18764=CARTESIAN_POINT('Ctrl Pts',(6.34720530709739,-3.06549796425185,5.57820768068278));
#18765=CARTESIAN_POINT('Ctrl Pts',(5.86953086171109,-3.04944298539597,5.64319531743515));
#18766=CARTESIAN_POINT('Ctrl Pts',(5.49584975715717,-3.17960634615903,5.69707450016525));
#18767=CARTESIAN_POINT('Ctrl Pts',(5.18167374083759,-3.48641160818447,5.75599838207982));
#18768=CARTESIAN_POINT('Ctrl Pts',(5.04197029026427,-3.94140910039868,5.81987647010874));
#18769=CARTESIAN_POINT('Ctrl Pts',(5.12029863594809,-4.32753826506529,5.87278413743482));
#18770=CARTESIAN_POINT('Ctrl Pts',(5.2663149982563,-4.55288629523623,5.90966649482064));
#18771=CARTESIAN_POINT('Ctrl Pts',(5.37117741816517,-4.66310330254181,5.93069699853573));
#18772=CARTESIAN_POINT('Ctrl Pts',(5.54752519184094,-4.80762211066538,5.96220176022617));
#18773=CARTESIAN_POINT('Ctrl Pts',(5.87417596723426,-4.93562642650329,6.00930677655604));
#18774=CARTESIAN_POINT('Ctrl Pts',(6.29769637485263,-4.88232598337754,6.06660612467952));
#18775=CARTESIAN_POINT('Ctrl Pts',(6.62047379630039,-4.67906087756066,6.11850395269178));
#18776=CARTESIAN_POINT('Ctrl Pts',(6.82362142151304,-4.4037527855136,6.16506694041442));
#18777=CARTESIAN_POINT('Ctrl Pts',(6.91192017974991,-4.07401150590665,6.21150986460091));
#18778=CARTESIAN_POINT('Ctrl Pts',(6.87373604354229,-3.73565491190597,6.25784046646843));
#18779=CARTESIAN_POINT('Ctrl Pts',(6.71481960446947,-3.43533167367221,6.3040764125896));
#18780=CARTESIAN_POINT('Ctrl Pts',(6.45774003972392,-3.21399047925324,6.35023076864715));
#18781=CARTESIAN_POINT('Ctrl Pts',(6.13801384513281,-3.10236364071456,6.39631970034203));
#18782=CARTESIAN_POINT('Ctrl Pts',(5.74348593015072,-3.11679890656582,6.45002812788936));
#18783=CARTESIAN_POINT('Ctrl Pts',(5.34012414260463,-3.33894846419464,6.51135232543338));
#18784=CARTESIAN_POINT('Ctrl Pts',(5.08970971672879,-3.79287801839994,6.5803109175142));
#18785=CARTESIAN_POINT('Ctrl Pts',(5.11394525582943,-4.22367302794002,6.63779297160539));
#18786=CARTESIAN_POINT('Ctrl Pts',(5.26859250522411,-4.52182198991263,6.68381562742008));
#18787=CARTESIAN_POINT('Ctrl Pts',(5.46062438052977,-4.72528715932241,6.7221950091176));
#18788=CARTESIAN_POINT('Ctrl Pts',(5.73533948531848,-4.87056941349058,6.76445662901709));
#18789=CARTESIAN_POINT('Ctrl Pts',(6.07241401329558,-4.90852365400217,6.81063041932966));
#18790=CARTESIAN_POINT('Ctrl Pts',(6.45585514108403,-4.80634676067811,6.8645984283862));
#18791=CARTESIAN_POINT('Ctrl Pts',(6.80245047206153,-4.49730107889992,6.92644266376476));
#18792=CARTESIAN_POINT('Ctrl Pts',(6.94792656407525,-3.99279744060583,6.99628588167397));
#18793=CARTESIAN_POINT('Ctrl Pts',(6.80243409723874,-3.48638510759692,7.06644845435211));
#18794=CARTESIAN_POINT('Ctrl Pts',(6.40764162124333,-3.13281085464808,7.13697136148438));
#18795=CARTESIAN_POINT('Ctrl Pts',(5.88234601693467,-3.04340282592901,7.20790251461747));
#18796=CARTESIAN_POINT('Ctrl Pts',(5.38671136540327,-3.24801639362842,7.27927901227808));
#18797=CARTESIAN_POINT('Ctrl Pts',(5.0740013431706,-3.68807082076264,7.35113797216885));
#18798=CARTESIAN_POINT('Ctrl Pts',(5.04267804088376,-4.2308763596221,7.42351167554797));
#18799=CARTESIAN_POINT('Ctrl Pts',(5.30731187114947,-4.71069600094691,7.49642855210674));
#18800=CARTESIAN_POINT('Ctrl Pts',(5.79029962646666,-4.97836689832941,7.56992328530873));
#18801=CARTESIAN_POINT('Ctrl Pts',(6.34616999591135,-4.94778675880538,7.6440187765564));
#18802=CARTESIAN_POINT('Ctrl Pts',(6.80455108078886,-4.62356423479621,7.71873312942426));
#18803=CARTESIAN_POINT('Ctrl Pts',(7.02159429958252,-4.10059489849228,7.79409235639335));
#18804=CARTESIAN_POINT('Ctrl Pts',(6.92677315546898,-3.53754527937747,7.87010761270296));
#18805=CARTESIAN_POINT('Ctrl Pts',(6.54335772488925,-3.10743806009348,7.94678244740374));
#18806=CARTESIAN_POINT('Ctrl Pts',(5.98529704655144,-2.94609162323264,8.02413006489736));
#18807=CARTESIAN_POINT('Ctrl Pts',(5.42164916618205,-3.10728509594054,8.10214039646089));
#18808=CARTESIAN_POINT('Ctrl Pts',(5.04202949373677,-3.53143448190436,8.17791337266471));
#18809=CARTESIAN_POINT('Ctrl Pts',(4.93356821182761,-4.06783639076264,8.2513417969401));
#18810=CARTESIAN_POINT('Ctrl Pts',(5.08862282161157,-4.57369791196422,8.32235735676531));
#18811=CARTESIAN_POINT('Ctrl Pts',(5.43823576048116,-4.91492383754914,8.38792025541212));
#18812=CARTESIAN_POINT('Ctrl Pts',(5.85433946781558,-5.06047867538894,8.44788715643451));
#18813=CARTESIAN_POINT('Ctrl Pts',(6.25271887238557,-5.04587511822749,8.50212325209872));
#18814=CARTESIAN_POINT('Ctrl Pts',(6.61999951562128,-4.88572034405795,8.55663424769427));
#18815=CARTESIAN_POINT('Ctrl Pts',(6.90476939932178,-4.60122727426364,8.61139993288472));
#18816=CARTESIAN_POINT('Ctrl Pts',(7.06665260714968,-4.23063194099307,8.66641839038366));
#18817=CARTESIAN_POINT('Ctrl Pts',(7.08200568370839,-3.82474181939741,8.72168000590468));
#18818=CARTESIAN_POINT('Ctrl Pts',(6.947433257179,-3.43967321822155,8.7771760282935));
#18819=CARTESIAN_POINT('Ctrl Pts',(6.68039689961518,-3.12914741165085,8.83289647602786));
#18820=CARTESIAN_POINT('Ctrl Pts',(6.31697702825656,-2.93691623733113,8.88883108316005));
#18821=CARTESIAN_POINT('Ctrl Pts',(5.90695860513133,-2.89059061296164,8.94496880460782));
#18822=CARTESIAN_POINT('Ctrl Pts',(5.50700490680685,-2.99762875074735,9.0012983390224));
#18823=CARTESIAN_POINT('Ctrl Pts',(5.17272540838232,-3.24419480617616,9.05780734478288));
#18824=CARTESIAN_POINT('Ctrl Pts',(4.95102157956017,-3.59685017820169,9.11448414857256));
#18825=CARTESIAN_POINT('Ctrl Pts',(4.87318814711464,-4.00732421615173,9.17131408794555));
#18826=CARTESIAN_POINT('Ctrl Pts',(4.95108701817399,-4.41868857022641,9.22828780042604));
#18827=CARTESIAN_POINT('Ctrl Pts',(5.19894039635913,-4.81381967302136,9.29173363197765));
#18828=CARTESIAN_POINT('Ctrl Pts',(5.63639590476303,-5.09688098930182,9.36168596521111));
#18829=CARTESIAN_POINT('Ctrl Pts',(6.20488341287629,-5.13929550996791,9.43816289043042));
#18830=CARTESIAN_POINT('Ctrl Pts',(6.60031943017411,-4.96097203670386,9.49642064148387));
#18831=CARTESIAN_POINT('Ctrl Pts',(6.8130702619607,-4.76504447047869,9.5363558838958));
#18832=CARTESIAN_POINT('Ctrl Pts',(6.94511802689851,-4.60412809383265,9.56511887960774));
#18833=CARTESIAN_POINT('Ctrl Pts',(7.11437864669289,-4.27798597899338,9.61547396389942));
#18834=CARTESIAN_POINT('Ctrl Pts',(7.14491779222484,-3.73829148440297,9.68745604502794));
#18835=CARTESIAN_POINT('Ctrl Pts',(6.83083864734627,-3.17009688337909,9.77385551909786));
#18836=CARTESIAN_POINT('Ctrl Pts',(6.26290699701676,-2.8562934070938,9.86022492860254));
#18837=CARTESIAN_POINT('Ctrl Pts',(5.61575197634126,-2.89286502547761,9.94651247809435));
#18838=CARTESIAN_POINT('Ctrl Pts',(5.08778619204425,-3.26729393662258,10.0326676206064));
#18839=CARTESIAN_POINT('Ctrl Pts',(4.84092188303821,-3.86424218979877,10.1186403336879));
#18840=CARTESIAN_POINT('Ctrl Pts',(4.94906070406917,-4.49919530585996,10.2043810035239));
#18841=CARTESIAN_POINT('Ctrl Pts',(5.37714255217191,-4.97773968110716,10.2898422024077));
#18842=CARTESIAN_POINT('Ctrl Pts',(5.99182700819212,-5.15443673839473,10.3749777902456));
#18843=CARTESIAN_POINT('Ctrl Pts',(6.6036286643445,-4.9777550601931,10.4597437013092));
#18844=CARTESIAN_POINT('Ctrl Pts',(7.02554665450114,-4.50493359335247,10.5440980117182));
#18845=CARTESIAN_POINT('Ctrl Pts',(7.13063227624352,-3.88344998774725,10.6280012139768));
#18846=CARTESIAN_POINT('Ctrl Pts',(6.890317183568,-3.30472348185151,10.7114166464371));
#18847=CARTESIAN_POINT('Ctrl Pts',(6.38212732946614,-2.9448499039503,10.7943101163743));
#18848=CARTESIAN_POINT('Ctrl Pts',(5.76446732461662,-2.9107896777846,10.8766515375219));
#18849=CARTESIAN_POINT('Ctrl Pts',(5.22726169429406,-3.20844365100958,10.958411932489));
#18850=CARTESIAN_POINT('Ctrl Pts',(4.93276927196662,-3.74240011088686,11.0395707404944));
#18851=CARTESIAN_POINT('Ctrl Pts',(4.96767361997263,-4.34631263085527,11.1201000860987));
#18852=CARTESIAN_POINT('Ctrl Pts',(5.31535533916341,-4.83541600550362,11.1999832745146));
#18853=CARTESIAN_POINT('Ctrl Pts',(5.86556113061819,-5.06246353418302,11.2792176122038));
#18854=CARTESIAN_POINT('Ctrl Pts',(6.44726148398534,-4.96317297736691,11.3577766442642));
#18855=CARTESIAN_POINT('Ctrl Pts',(6.88312582385536,-4.57225455833006,11.4356903944807));
#18856=CARTESIAN_POINT('Ctrl Pts',(6.98969410226672,-4.20147268401305,11.4871431260612));
#18857=CARTESIAN_POINT('Ctrl Pts',(6.98971912848012,-4.01557182757373,11.5128070631624));
#18858=CARTESIAN_POINT('Ctrl Pts',(7.02991808875672,-3.9863204986747,2.60093950625054));
#18859=CARTESIAN_POINT('Ctrl Pts',(7.0298920767563,-3.79309660190507,2.62761440178745));
#18860=CARTESIAN_POINT('Ctrl Pts',(6.91909382179967,-3.40769064837915,2.68109050706102));
#18861=CARTESIAN_POINT('Ctrl Pts',(6.46676608976936,-3.00219879487548,2.76192331287528));
#18862=CARTESIAN_POINT('Ctrl Pts',(5.86416835249228,-2.89947315565633,2.84329274697736));
#18863=CARTESIAN_POINT('Ctrl Pts',(5.29547823170544,-3.13436399239426,2.92520207327125));
#18864=CARTESIAN_POINT('Ctrl Pts',(4.93671383355777,-3.63910836719776,3.00761460452821));
#18865=CARTESIAN_POINT('Ctrl Pts',(4.90144022313547,-4.26079346404597,3.09050869847464));
#18866=CARTESIAN_POINT('Ctrl Pts',(5.20362252301616,-4.80919944690218,3.17384785225833));
#18867=CARTESIAN_POINT('Ctrl Pts',(5.75431021582355,-5.11388475786273,3.25759644032169));
#18868=CARTESIAN_POINT('Ctrl Pts',(6.38540320153558,-5.07886240663714,3.34172581662129));
#18869=CARTESIAN_POINT('Ctrl Pts',(6.90325242066822,-4.71186766302553,3.42619408052645));
#18870=CARTESIAN_POINT('Ctrl Pts',(7.14727039378041,-4.12354721671033,3.51096234986392));
#18871=CARTESIAN_POINT('Ctrl Pts',(7.04052980174623,-3.49366540997803,3.59598782843037));
#18872=CARTESIAN_POINT('Ctrl Pts',(6.61390657684921,-3.01594762654595,3.6812269984434));
#18873=CARTESIAN_POINT('Ctrl Pts',(5.9973096813911,-2.83814561164906,3.76663507596031));
#18874=CARTESIAN_POINT('Ctrl Pts',(5.37968234307175,-3.01590762291788,3.85216530550586));
#18875=CARTESIAN_POINT('Ctrl Pts',(4.96698506179213,-3.47783712150818,3.9346017628615));
#18876=CARTESIAN_POINT('Ctrl Pts',(4.86906342867886,-3.96439384809991,4.0012048778156));
#18877=CARTESIAN_POINT('Ctrl Pts',(4.92546013389047,-4.28269662274511,4.04560996804786));
#18878=CARTESIAN_POINT('Ctrl Pts',(4.990412763925,-4.45442047509628,4.07098315160127));
#18879=CARTESIAN_POINT('Ctrl Pts',(5.11895625152796,-4.6979784138749,4.10903845085798));
#18880=CARTESIAN_POINT('Ctrl Pts',(5.42317137440073,-4.99492329369231,4.16607662934805));
#18881=CARTESIAN_POINT('Ctrl Pts',(5.968352558652,-5.14822243535607,4.2420839301269));
#18882=CARTESIAN_POINT('Ctrl Pts',(6.51978304095379,-5.02234952447351,4.31797503338202));
#18883=CARTESIAN_POINT('Ctrl Pts',(6.9072832001042,-4.67955144327851,4.38740393573842));
#18884=CARTESIAN_POINT('Ctrl Pts',(7.09212835650512,-4.25495690058516,4.45041049887341));
#18885=CARTESIAN_POINT('Ctrl Pts',(7.10785181269314,-3.83924601052615,4.50699939833727));
#18886=CARTESIAN_POINT('Ctrl Pts',(6.97044503028521,-3.44765854135089,4.56346997832381));
#18887=CARTESIAN_POINT('Ctrl Pts',(6.67054717410501,-3.09855890921501,4.62606392322435));
#18888=CARTESIAN_POINT('Ctrl Pts',(6.20426157743975,-2.88844544026138,4.69471395250901));
#18889=CARTESIAN_POINT('Ctrl Pts',(5.64980765832729,-2.9303193519752,4.76932248356804));
#18890=CARTESIAN_POINT('Ctrl Pts',(5.2820875278432,-3.16834842314897,4.82810745942499));
#18891=CARTESIAN_POINT('Ctrl Pts',(5.09152989701439,-3.41718119774718,4.87131005699247));
#18892=CARTESIAN_POINT('Ctrl Pts',(4.97054323829609,-3.65648857388211,4.9082745060722));
#18893=CARTESIAN_POINT('Ctrl Pts',(4.90764740745214,-3.98932272899894,4.95435456202079));
#18894=CARTESIAN_POINT('Ctrl Pts',(4.98320524804316,-4.38709184426172,5.00944034588392));
#18895=CARTESIAN_POINT('Ctrl Pts',(5.19781986825172,-4.72860825805215,5.06430729650093));
#18896=CARTESIAN_POINT('Ctrl Pts',(5.52108471179064,-4.96679238484029,5.11894800494866));
#18897=CARTESIAN_POINT('Ctrl Pts',(5.90757483068251,-5.07041839122686,5.17335835282008));
#18898=CARTESIAN_POINT('Ctrl Pts',(6.30287112434244,-5.02533471611233,5.22752888227952));
#18899=CARTESIAN_POINT('Ctrl Pts',(6.77118875319483,-4.77916066880441,5.29943161761435));
#18900=CARTESIAN_POINT('Ctrl Pts',(7.11631632438462,-4.18127802959054,5.3886627139529));
#18901=CARTESIAN_POINT('Ctrl Pts',(6.93160691706252,-3.3792984463582,5.49470538718602));
#18902=CARTESIAN_POINT('Ctrl Pts',(6.37115716117766,-3.00004224169406,5.58217557531111));
#18903=CARTESIAN_POINT('Ctrl Pts',(5.86067088430187,-2.98290615431278,5.6516158762443));
#18904=CARTESIAN_POINT('Ctrl Pts',(5.46137234532083,-3.12199756637258,5.70918062040184));
#18905=CARTESIAN_POINT('Ctrl Pts',(5.12579786574395,-3.44975370223118,5.77211265498338));
#18906=CARTESIAN_POINT('Ctrl Pts',(4.97675035295965,-3.93542942576474,5.84028080193706));
#18907=CARTESIAN_POINT('Ctrl Pts',(5.06033761012733,-4.34715442903143,5.89669313304848));
#18908=CARTESIAN_POINT('Ctrl Pts',(5.21589312480973,-4.58717538667364,5.93597358008697));
#18909=CARTESIAN_POINT('Ctrl Pts',(5.32753388253116,-4.70451276882046,5.95836231407345));
#18910=CARTESIAN_POINT('Ctrl Pts',(5.51520437334612,-4.85830387801752,5.9918868858073));
#18911=CARTESIAN_POINT('Ctrl Pts',(5.86247379692578,-4.99428552612942,6.0419557148591));
#18912=CARTESIAN_POINT('Ctrl Pts',(6.31174700962642,-4.93760907536453,6.10273651590458));
#18913=CARTESIAN_POINT('Ctrl Pts',(6.65339834000255,-4.72234495572188,6.15767095052905));
#18914=CARTESIAN_POINT('Ctrl Pts',(6.8679953212426,-4.43140295203578,6.20687048242351));
#18915=CARTESIAN_POINT('Ctrl Pts',(6.96101113211587,-4.08370529584463,6.25583653383823));
#18916=CARTESIAN_POINT('Ctrl Pts',(6.92075607352957,-3.72776957037704,6.30457519859578));
#18917=CARTESIAN_POINT('Ctrl Pts',(6.75390517552733,-3.41265101808349,6.35309493042986));
#18918=CARTESIAN_POINT('Ctrl Pts',(6.48475640607782,-3.18104900332911,6.40140514207317));
#18919=CARTESIAN_POINT('Ctrl Pts',(6.15098997417316,-3.06462900410609,6.44951457052472));
#18920=CARTESIAN_POINT('Ctrl Pts',(5.74035948083984,-3.0797743123596,6.50541569711097));
#18921=CARTESIAN_POINT('Ctrl Pts',(5.32224947191523,-3.31042394608842,6.5690097802638));
#18922=CARTESIAN_POINT('Ctrl Pts',(5.0641868258842,-3.77904585095687,6.64017852499677));
#18923=CARTESIAN_POINT('Ctrl Pts',(5.0893877649522,-4.22134632032621,6.6992024061301));
#18924=CARTESIAN_POINT('Ctrl Pts',(5.24761803700627,-4.52623489545367,6.74627803713346));
#18925=CARTESIAN_POINT('Ctrl Pts',(5.44354313111177,-4.73374792005069,6.78543039430136));
#18926=CARTESIAN_POINT('Ctrl Pts',(5.72295852635408,-4.88138222484995,6.82841428842587));
#18927=CARTESIAN_POINT('Ctrl Pts',(6.06447743648484,-4.91972128359138,6.87519838300688));
#18928=CARTESIAN_POINT('Ctrl Pts',(6.45152349101931,-4.81642569389462,6.92968667403752));
#18929=CARTESIAN_POINT('Ctrl Pts',(6.79954537293466,-4.50562749044762,6.99183260293409));
#18930=CARTESIAN_POINT('Ctrl Pts',(6.94448755821497,-4.00135704634088,7.06165092921972));
#18931=CARTESIAN_POINT('Ctrl Pts',(6.79951105295416,-3.49822641785881,7.13139191346124));
#18932=CARTESIAN_POINT('Ctrl Pts',(6.40903366533783,-3.14907814500179,7.20111945270289));
#18933=CARTESIAN_POINT('Ctrl Pts',(5.89262195791797,-3.06157288901472,7.27085739388313));
#18934=CARTESIAN_POINT('Ctrl Pts',(5.40812254199752,-3.26200851208852,7.34066372988413));
#18935=CARTESIAN_POINT('Ctrl Pts',(5.10418067172973,-3.69034738245555,7.41058819563509));
#18936=CARTESIAN_POINT('Ctrl Pts',(5.07421407730807,-4.21594541569564,7.48068129780375));
#18937=CARTESIAN_POINT('Ctrl Pts',(5.32958846913487,-4.67828762483568,7.55099734167383));
#18938=CARTESIAN_POINT('Ctrl Pts',(5.79329453600511,-4.93490538629606,7.62156008648381));
#18939=CARTESIAN_POINT('Ctrl Pts',(6.32466741939653,-4.90539161700316,7.69241833598134));
#18940=CARTESIAN_POINT('Ctrl Pts',(6.7611327378177,-4.59633338526078,7.763618222302));
#18941=CARTESIAN_POINT('Ctrl Pts',(6.96696593812447,-4.09977663923876,7.83517991770188));
#18942=CARTESIAN_POINT('Ctrl Pts',(6.87700234449016,-3.56684830698183,7.90714553328152));
#18943=CARTESIAN_POINT('Ctrl Pts',(6.51484228409451,-3.16087025594183,7.97956166490427));
#18944=CARTESIAN_POINT('Ctrl Pts',(5.98902418310519,-3.00899219730746,8.05244618048738));
#18945=CARTESIAN_POINT('Ctrl Pts',(5.45889377764469,-3.16073805954472,8.12584776997905));
#18946=CARTESIAN_POINT('Ctrl Pts',(5.10240229055434,-3.55916285129593,8.19702745975862));
#18947=CARTESIAN_POINT('Ctrl Pts',(5.00063529264588,-4.06258448759413,8.26596672294065));
#18948=CARTESIAN_POINT('Ctrl Pts',(5.14608638641085,-4.5370310753527,8.33258570888342));
#18949=CARTESIAN_POINT('Ctrl Pts',(5.47390473949641,-4.85700122338878,8.39407564739306));
#18950=CARTESIAN_POINT('Ctrl Pts',(5.86409370988404,-4.99349801167686,8.45031426874171));
#18951=CARTESIAN_POINT('Ctrl Pts',(6.23778180866483,-4.97982005074953,8.5012050843239));
#18952=CARTESIAN_POINT('Ctrl Pts',(6.5824024810436,-4.82957017385029,8.55235608559697));
#18953=CARTESIAN_POINT('Ctrl Pts',(6.84977764807081,-4.56249579195602,8.60378338768071));
#18954=CARTESIAN_POINT('Ctrl Pts',(7.0018975831038,-4.2143396128522,8.6554816689866));
#18955=CARTESIAN_POINT('Ctrl Pts',(7.01637606498482,-3.83268836849798,8.7074523074285));
#18956=CARTESIAN_POINT('Ctrl Pts',(6.88975870622095,-3.47023825895862,8.75969440257842));
#18957=CARTESIAN_POINT('Ctrl Pts',(6.63817267282148,-3.17759763612041,8.81220696108591));
#18958=CARTESIAN_POINT('Ctrl Pts',(6.29531438742434,-2.99617683490492,8.86498799953351));
#18959=CARTESIAN_POINT('Ctrl Pts',(5.90792353151983,-2.95234443557854,8.91803494390907));
#18960=CARTESIAN_POINT('Ctrl Pts',(5.52943465947779,-3.05356766071865,8.9713444776914));
#18961=CARTESIAN_POINT('Ctrl Pts',(5.21253830696404,-3.28722085945642,9.02491258570221));
#18962=CARTESIAN_POINT('Ctrl Pts',(5.00195199494555,-3.62204646733453,9.07873463013611));
#18963=CARTESIAN_POINT('Ctrl Pts',(4.92781914311232,-4.01254248071306,9.13280515564705));
#18964=CARTESIAN_POINT('Ctrl Pts',(5.00199615651236,-4.40470108927855,9.18711842200491));
#18965=CARTESIAN_POINT('Ctrl Pts',(5.23867881713171,-4.78221302009702,9.24772886990218));
#18966=CARTESIAN_POINT('Ctrl Pts',(5.65754135413719,-5.05347587134047,9.31472611241896));
#18967=CARTESIAN_POINT('Ctrl Pts',(6.20369084805172,-5.09446619773149,9.38820047058106));
#18968=CARTESIAN_POINT('Ctrl Pts',(6.58491140028356,-4.9227463833809,9.44435213091082));
#18969=CARTESIAN_POINT('Ctrl Pts',(6.79043706915131,-4.73349491889994,9.48292799960354));
#18970=CARTESIAN_POINT('Ctrl Pts',(6.91812074774067,-4.57790769275921,9.51073873753964));
#18971=CARTESIAN_POINT('Ctrl Pts',(7.08206628048093,-4.26214523314509,9.55949576991338));
#18972=CARTESIAN_POINT('Ctrl Pts',(7.11203000974648,-3.73801507749313,9.62940143023879));
#18973=CARTESIAN_POINT('Ctrl Pts',(6.80607956694539,-3.18372878894946,9.71365355088675));
#18974=CARTESIAN_POINT('Ctrl Pts',(6.2500729387616,-2.87606410279642,9.79823196594816));
#18975=CARTESIAN_POINT('Ctrl Pts',(5.61350827590933,-2.91164276328602,9.88309878900258));
#18976=CARTESIAN_POINT('Ctrl Pts',(5.09167653337187,-3.28121508261429,9.96820541651057));
#18977=CARTESIAN_POINT('Ctrl Pts',(4.84631772029848,-3.87343097145342,10.053501888748));
#18978=CARTESIAN_POINT('Ctrl Pts',(4.95370265231542,-4.50645428090226,10.1389580152242));
#18979=CARTESIAN_POINT('Ctrl Pts',(5.38206584333841,-4.98594004162619,10.224520377509));
#18980=CARTESIAN_POINT('Ctrl Pts',(6.00029102821274,-5.16409124961399,10.310145146497));
#18981=CARTESIAN_POINT('Ctrl Pts',(6.61864143146891,-4.9859514705061,10.395783712958));
#18982=CARTESIAN_POINT('Ctrl Pts',(7.04722318405374,-4.50628003310617,10.4813893153194));
#18983=CARTESIAN_POINT('Ctrl Pts',(7.15476578245007,-3.87269332662491,10.5669147992673));
#18984=CARTESIAN_POINT('Ctrl Pts',(6.90903852094291,-3.27989871424364,10.6523132378576));
#18985=CARTESIAN_POINT('Ctrl Pts',(6.38662842519509,-2.909479749711,10.7375396128794));
#18986=CARTESIAN_POINT('Ctrl Pts',(5.7487891451485,-2.87392013799551,10.8225468482879));
#18987=CARTESIAN_POINT('Ctrl Pts',(5.19161128486125,-3.18222383349236,10.9072959154668));
#18988=CARTESIAN_POINT('Ctrl Pts',(4.88477218880103,-3.7377854487073,10.991733743207));
#18989=CARTESIAN_POINT('Ctrl Pts',(4.92090890603324,-4.36871687716726,11.0758429802562));
#18990=CARTESIAN_POINT('Ctrl Pts',(5.28513006682729,-4.8816390523311,11.1595745791957));
#18991=CARTESIAN_POINT('Ctrl Pts',(5.86367097478207,-5.12070465769319,11.2428883860081));
#18992=CARTESIAN_POINT('Ctrl Pts',(6.47730091809014,-5.01618325405715,11.3257454113017));
#18993=CARTESIAN_POINT('Ctrl Pts',(6.93846782961665,-4.60290035590192,11.4081371563723));
#18994=CARTESIAN_POINT('Ctrl Pts',(7.05150181122088,-4.20962129145193,11.4626969504376));
#18995=CARTESIAN_POINT('Ctrl Pts',(7.05152835862385,-4.01242066548927,11.4899208404075));
#18996=CARTESIAN_POINT('Ctrl Pts',(6.99999815899365,-3.98632452652653,2.60093950625054));
#18997=CARTESIAN_POINT('Ctrl Pts',(6.99997288064459,-3.79855038269031,2.62686205390176));
#18998=CARTESIAN_POINT('Ctrl Pts',(6.89233514047511,-3.42414397295474,2.67881370715146));
#18999=CARTESIAN_POINT('Ctrl Pts',(6.45271448161715,-3.02998089899105,2.757384351524));
#19000=CARTESIAN_POINT('Ctrl Pts',(5.86671979479608,-2.93006055988124,2.83651312593273));
#19001=CARTESIAN_POINT('Ctrl Pts',(5.31329781017118,-3.15858496371257,2.91622300969429));
#19002=CARTESIAN_POINT('Ctrl Pts',(4.9638387202763,-3.65012742948249,2.99648818069946));
#19003=CARTESIAN_POINT('Ctrl Pts',(4.9293710419426,-4.25616717719541,3.07729927110974));
#19004=CARTESIAN_POINT('Ctrl Pts',(5.22419213535424,-4.79140012919127,3.15863486906283));
#19005=CARTESIAN_POINT('Ctrl Pts',(5.76222069265107,-5.08919945404236,3.24047453667969));
#19006=CARTESIAN_POINT('Ctrl Pts',(6.379677030618,-5.05504702300603,3.32279319426342));
#19007=CARTESIAN_POINT('Ctrl Pts',(6.88712884688249,-4.6955749219134,3.40556355651458));
#19008=CARTESIAN_POINT('Ctrl Pts',(7.12670085302573,-4.11831918936923,3.48875539197247));
#19009=CARTESIAN_POINT('Ctrl Pts',(7.02192637673817,-3.49920475943206,3.57233609217612));
#19010=CARTESIAN_POINT('Ctrl Pts',(6.60200480535371,-3.02877356919622,3.65627071403784));
#19011=CARTESIAN_POINT('Ctrl Pts',(5.99389696970595,-2.85326346917548,3.74052223770667));
#19012=CARTESIAN_POINT('Ctrl Pts',(5.38356210524816,-3.02876561374954,3.82505176545516));
#19013=CARTESIAN_POINT('Ctrl Pts',(4.97486808401256,-3.48597581907603,3.90667922332894));
#19014=CARTESIAN_POINT('Ctrl Pts',(4.87764331063032,-3.96854834063101,3.97275270796177));
#19015=CARTESIAN_POINT('Ctrl Pts',(4.93363491104256,-4.28466096216571,4.01685604464165));
#19016=CARTESIAN_POINT('Ctrl Pts',(4.99817931143911,-4.45530970670709,4.04207155735716));
#19017=CARTESIAN_POINT('Ctrl Pts',(5.12597275373369,-4.69744865131441,4.07990746653167));
#19018=CARTESIAN_POINT('Ctrl Pts',(5.42875069944469,-4.99309340796393,4.13670511444809));
#19019=CARTESIAN_POINT('Ctrl Pts',(5.97231920216535,-5.14605898976926,4.21249748606625));
#19020=CARTESIAN_POINT('Ctrl Pts',(6.52320508223107,-5.02044374257342,4.28832048254892));
#19021=CARTESIAN_POINT('Ctrl Pts',(6.91110467076896,-4.67743260856581,4.35782392841035));
#19022=CARTESIAN_POINT('Ctrl Pts',(7.09644745188598,-4.25185787791867,4.42098501720712));
#19023=CARTESIAN_POINT('Ctrl Pts',(7.11227598252982,-3.83457932502243,4.47779828333078));
#19024=CARTESIAN_POINT('Ctrl Pts',(6.97422198867159,-3.44096105119827,4.53456659991209));
#19025=CARTESIAN_POINT('Ctrl Pts',(6.67241777459347,-3.08955752755044,4.59757801617794));
#19026=CARTESIAN_POINT('Ctrl Pts',(6.20242890124212,-2.8776477149725,4.66678930738527));
#19027=CARTESIAN_POINT('Ctrl Pts',(5.64251878205079,-2.91980762281901,4.74213608937642));
#19028=CARTESIAN_POINT('Ctrl Pts',(5.2704159386044,-3.1605530148329,4.80163845364204));
#19029=CARTESIAN_POINT('Ctrl Pts',(5.0774166278585,-3.41255654376288,4.84539629257686));
#19030=CARTESIAN_POINT('Ctrl Pts',(4.95479769651029,-3.65506677262475,4.88286085266752));
#19031=CARTESIAN_POINT('Ctrl Pts',(4.89096164216428,-3.99267527518354,4.9296088561907));
#19032=CARTESIAN_POINT('Ctrl Pts',(4.9676452372308,-4.39667000889553,4.98556279567646));
#19033=CARTESIAN_POINT('Ctrl Pts',(5.18583996189851,-4.74396038265063,5.04136211338706));
#19034=CARTESIAN_POINT('Ctrl Pts',(5.51489715544512,-4.98648283834255,5.09699623582978));
#19035=CARTESIAN_POINT('Ctrl Pts',(5.90877797642046,-5.0921366099034,5.15245506500268));
#19036=CARTESIAN_POINT('Ctrl Pts',(6.31208382647452,-5.04618505638536,5.20772889790527));
#19037=CARTESIAN_POINT('Ctrl Pts',(6.79039563711824,-4.79482787477752,5.28116853494519));
#19038=CARTESIAN_POINT('Ctrl Pts',(7.14364250607538,-4.18339760328549,5.37246079320281));
#19039=CARTESIAN_POINT('Ctrl Pts',(6.95465392442801,-3.3615290602033,5.48113680479085));
#19040=CARTESIAN_POINT('Ctrl Pts',(6.37954281770185,-2.97211167108618,5.57092649504958));
#19041=CARTESIAN_POINT('Ctrl Pts',(5.85508217241069,-2.95446460563552,5.64227218334414));
#19042=CARTESIAN_POINT('Ctrl Pts',(5.44460306454923,-3.0974244576334,5.70145206942602));
#19043=CARTESIAN_POINT('Ctrl Pts',(5.09938139322235,-3.43453521092238,5.76619150122483));
#19044=CARTESIAN_POINT('Ctrl Pts',(4.94592320318296,-3.93442474869926,5.83636208316637));
#19045=CARTESIAN_POINT('Ctrl Pts',(5.03197265676116,-4.35840627465708,5.89445465107149));
#19046=CARTESIAN_POINT('Ctrl Pts',(5.19219264369348,-4.60564299044654,5.93491706685731));
#19047=CARTESIAN_POINT('Ctrl Pts',(5.30719577297855,-4.72651611720447,5.95798055540973));
#19048=CARTESIAN_POINT('Ctrl Pts',(5.50053046023923,-4.88495348501329,5.99251787759586));
#19049=CARTESIAN_POINT('Ctrl Pts',(5.85832951556707,-5.02507253962729,6.04410658286047));
#19050=CARTESIAN_POINT('Ctrl Pts',(6.32126493019694,-4.96668267597821,6.10673564915363));
#19051=CARTESIAN_POINT('Ctrl Pts',(6.67328517320073,-4.74489735077078,6.1633365491453));
#19052=CARTESIAN_POINT('Ctrl Pts',(6.89435900913716,-4.44516759248262,6.21402149084589));
#19053=CARTESIAN_POINT('Ctrl Pts',(6.99016055458223,-4.08705298460299,6.26445344730346));
#19054=CARTESIAN_POINT('Ctrl Pts',(6.94870527391535,-3.72056310115263,6.31463598339954));
#19055=CARTESIAN_POINT('Ctrl Pts',(6.77696548585144,-3.39623351183634,6.36457330966794));
#19056=CARTESIAN_POINT('Ctrl Pts',(6.50006848678236,-3.15797695360399,6.41427030439494));
#19057=CARTESIAN_POINT('Ctrl Pts',(6.15689079921747,-3.03828948600061,6.46373243937456));
#19058=CARTESIAN_POINT('Ctrl Pts',(5.73494713487383,-3.05387392617641,6.52117143017342));
#19059=CARTESIAN_POINT('Ctrl Pts',(5.30575107583077,-3.29070893773119,6.58644590514151));
#19060=CARTESIAN_POINT('Ctrl Pts',(5.04125313845857,-3.77122732190886,6.6594050878354));
#19061=CARTESIAN_POINT('Ctrl Pts',(5.06714113786846,-4.2240700226978,6.71983222627245));
#19062=CARTESIAN_POINT('Ctrl Pts',(5.22896371026909,-4.53583531846688,6.76796591127916));
#19063=CARTESIAN_POINT('Ctrl Pts',(5.42916113979845,-4.74785467675554,6.80796630808184));
#19064=CARTESIAN_POINT('Ctrl Pts',(5.714367370309,-4.89850759732021,6.85183024025803));
#19065=CARTESIAN_POINT('Ctrl Pts',(6.06253639457921,-4.93755475445945,6.89952195690528));
#19066=CARTESIAN_POINT('Ctrl Pts',(6.4565847787629,-4.83233977440753,6.95498839066731));
#19067=CARTESIAN_POINT('Ctrl Pts',(6.81022730237302,-4.51633849133825,7.01814871600544));
#19068=CARTESIAN_POINT('Ctrl Pts',(6.95706828830077,-4.00489886911992,7.08893287981098));
#19069=CARTESIAN_POINT('Ctrl Pts',(6.81021224891959,-3.49584469103884,7.15948666255227));
#19070=CARTESIAN_POINT('Ctrl Pts',(6.41592301667082,-3.14352189275395,7.22985222727915));
#19071=CARTESIAN_POINT('Ctrl Pts',(5.89582428767248,-3.0555832223308,7.30007283378182));
#19072=CARTESIAN_POINT('Ctrl Pts',(5.40914881608276,-3.25711226719962,7.37019262219717));
#19073=CARTESIAN_POINT('Ctrl Pts',(5.10471600640629,-3.68647088534127,7.4402563254545));
#19074=CARTESIAN_POINT('Ctrl Pts',(5.07493689936822,-4.21187381141773,7.51030900528994));
#19075=CARTESIAN_POINT('Ctrl Pts',(5.32972438815395,-4.67276168571651,7.58039577687912));
#19076=CARTESIAN_POINT('Ctrl Pts',(5.79102554371443,-4.92784792737786,7.65056157421906));
#19077=CARTESIAN_POINT('Ctrl Pts',(6.31826031255578,-4.89837953861158,7.72085085714204));
#19078=CARTESIAN_POINT('Ctrl Pts',(6.75020660471299,-4.59231290695902,7.79130734550421));
#19079=CARTESIAN_POINT('Ctrl Pts',(6.95334524231267,-4.10180979072915,7.86197377515194));
#19080=CARTESIAN_POINT('Ctrl Pts',(6.86452811856373,-3.57660445666216,7.93289164673106));
#19081=CARTESIAN_POINT('Ctrl Pts',(6.50822949801913,-3.17741851765368,8.00410096472273));
#19082=CARTESIAN_POINT('Ctrl Pts',(5.99202912111436,-3.02846879700038,8.07564001126929));
#19083=CARTESIAN_POINT('Ctrl Pts',(5.47262775862424,-3.1772786287127,8.14754510192845));
#19084=CARTESIAN_POINT('Ctrl Pts',(5.12396773984527,-3.56713104102442,8.21717245978697));
#19085=CARTESIAN_POINT('Ctrl Pts',(5.02465088008016,-4.0589090579052,8.28449962671212));
#19086=CARTESIAN_POINT('Ctrl Pts',(5.16664179671633,-4.52183049710153,8.34949563002517));
#19087=CARTESIAN_POINT('Ctrl Pts',(5.48622133819085,-4.83366725020512,8.40942447534479));
#19088=CARTESIAN_POINT('Ctrl Pts',(5.86625745021743,-4.9665851067969,8.4641954747342));
#19089=CARTESIAN_POINT('Ctrl Pts',(6.22997586892847,-4.95324406413884,8.5137197914407));
#19090=CARTESIAN_POINT('Ctrl Pts',(6.56523678307791,-4.80705258085916,8.56348049146453));
#19091=CARTESIAN_POINT('Ctrl Pts',(6.8252178463785,-4.54733568382595,8.61348288991823));
#19092=CARTESIAN_POINT('Ctrl Pts',(6.97306928054101,-4.20890471076454,8.6637316832973));
#19093=CARTESIAN_POINT('Ctrl Pts',(6.98712341108126,-3.83802816814003,8.7142309149468));
#19094=CARTESIAN_POINT('Ctrl Pts',(6.86409431800442,-3.4858887373625,8.76498396878373));
#19095=CARTESIAN_POINT('Ctrl Pts',(6.61968641501593,-3.20161333099039,8.81599356080702));
#19096=CARTESIAN_POINT('Ctrl Pts',(6.28663539552411,-3.02539046352671,8.8672617337013));
#19097=CARTESIAN_POINT('Ctrl Pts',(5.91032079687008,-2.98281618785264,8.9187898484193));
#19098=CARTESIAN_POINT('Ctrl Pts',(5.54261902100133,-3.08115683102349,8.97057858319571));
#19099=CARTESIAN_POINT('Ctrl Pts',(5.23470149593991,-3.30818973404657,9.02262792887906));
#19100=CARTESIAN_POINT('Ctrl Pts',(5.03002953653242,-3.63360637314209,9.07493719454492));
#19101=CARTESIAN_POINT('Ctrl Pts',(4.95795339049146,-4.01324887545392,9.12750499722226));
#19102=CARTESIAN_POINT('Ctrl Pts',(5.03008733681497,-4.39465616925505,9.18032929191999));
#19103=CARTESIAN_POINT('Ctrl Pts',(5.26037098227884,-4.76198737973904,9.23930488376548));
#19104=CARTESIAN_POINT('Ctrl Pts',(5.66815402132354,-5.02611715334513,9.30453505328307));
#19105=CARTESIAN_POINT('Ctrl Pts',(6.20031175950905,-5.06610553161693,9.37613052247429));
#19106=CARTESIAN_POINT('Ctrl Pts',(6.57211483447548,-4.89867154701958,9.43089482659667));
#19107=CARTESIAN_POINT('Ctrl Pts',(6.77268428325753,-4.71398594666241,9.46854124254023));
#19108=CARTESIAN_POINT('Ctrl Pts',(6.89732261541234,-4.56210906285714,9.4956893772699));
#19109=CARTESIAN_POINT('Ctrl Pts',(7.05743952416135,-4.25373892219051,9.54330952558428));
#19110=CARTESIAN_POINT('Ctrl Pts',(7.08681427060224,-3.7413976498585,9.61164803498953));
#19111=CARTESIAN_POINT('Ctrl Pts',(6.78743967682059,-3.19877575055479,9.69412425474241));
#19112=CARTESIAN_POINT('Ctrl Pts',(6.24245837315985,-2.89706443193603,9.77704206668623));
#19113=CARTESIAN_POINT('Ctrl Pts',(5.61746900273164,-2.93185417099466,9.86037047868398));
#19114=CARTESIAN_POINT('Ctrl Pts',(5.1042042416184,-3.29518411512121,9.94407604361117));
#19115=CARTESIAN_POINT('Ctrl Pts',(4.86233946758306,-3.8785536270643,10.0281231251224));
#19116=CARTESIAN_POINT('Ctrl Pts',(4.96816269898698,-4.50332086698013,10.1124740074888));
#19117=CARTESIAN_POINT('Ctrl Pts',(5.3915816199262,-4.97752738430232,10.1970892227568));
#19118=CARTESIAN_POINT('Ctrl Pts',(6.00397807691952,-5.15417755509278,10.281927720062));
#19119=CARTESIAN_POINT('Ctrl Pts',(6.61779621608409,-4.97752665860305,10.3669471357688));
#19120=CARTESIAN_POINT('Ctrl Pts',(7.04418758947222,-4.50057596349951,10.4521040140405));
#19121=CARTESIAN_POINT('Ctrl Pts',(7.15154318711507,-3.86917823804319,10.5373541207604));
#19122=CARTESIAN_POINT('Ctrl Pts',(6.9063217242137,-3.27712490715728,10.622652644332));
#19123=CARTESIAN_POINT('Ctrl Pts',(6.38365961018741,-2.90630232377856,10.70795449752));
#19124=CARTESIAN_POINT('Ctrl Pts',(5.74407957751689,-2.87046702674317,10.7932145497474));
#19125=CARTESIAN_POINT('Ctrl Pts',(5.18413779010185,-3.18009512220889,10.8783879953558));
#19126=CARTESIAN_POINT('Ctrl Pts',(4.87504525063398,-3.73939474085648,10.9634303821887));
#19127=CARTESIAN_POINT('Ctrl Pts',(4.9113280193628,-4.37593360867611,11.0482983399598));
#19128=CARTESIAN_POINT('Ctrl Pts',(5.27937248430205,-4.89450749674953,11.1329488708158));
#19129=CARTESIAN_POINT('Ctrl Pts',(5.86527624347711,-5.13679808752952,11.2173417295453));
#19130=CARTESIAN_POINT('Ctrl Pts',(6.48799534199112,-5.03087191620999,11.3014349903219));
#19131=CARTESIAN_POINT('Ctrl Pts',(6.95693136473707,-4.61090781293032,11.3851957485584));
#19132=CARTESIAN_POINT('Ctrl Pts',(7.07219562678886,-4.21035033769926,11.4407823887657));
#19133=CARTESIAN_POINT('Ctrl Pts',(7.07222266979228,-4.00946826992833,11.4685145081909));
#19134=CARTESIAN_POINT('',(6.99999815899365,-3.98632452652653,2.60093950625054));
#19135=CARTESIAN_POINT('Origin',(7.,-4.,2.7));
#19136=CARTESIAN_POINT('',(7.07222266979228,-4.00946826992833,11.4685145081909));
#19137=CARTESIAN_POINT('Ctrl Pts',(6.99999815899365,-3.98632452652653,2.60093950625054));
#19138=CARTESIAN_POINT('Ctrl Pts',(6.99997288064459,-3.79855038269031,2.62686205390176));
#19139=CARTESIAN_POINT('Ctrl Pts',(6.89233514047511,-3.42414397295474,2.67881370715146));
#19140=CARTESIAN_POINT('Ctrl Pts',(6.45271448161715,-3.02998089899105,2.757384351524));
#19141=CARTESIAN_POINT('Ctrl Pts',(5.86671979479608,-2.93006055988124,2.83651312593273));
#19142=CARTESIAN_POINT('Ctrl Pts',(5.31329781017118,-3.15858496371257,2.91622300969429));
#19143=CARTESIAN_POINT('Ctrl Pts',(4.9638387202763,-3.65012742948249,2.99648818069946));
#19144=CARTESIAN_POINT('Ctrl Pts',(4.9293710419426,-4.25616717719541,3.07729927110974));
#19145=CARTESIAN_POINT('Ctrl Pts',(5.22419213535424,-4.79140012919127,3.15863486906283));
#19146=CARTESIAN_POINT('Ctrl Pts',(5.76222069265107,-5.08919945404236,3.24047453667969));
#19147=CARTESIAN_POINT('Ctrl Pts',(6.379677030618,-5.05504702300603,3.32279319426342));
#19148=CARTESIAN_POINT('Ctrl Pts',(6.88712884688249,-4.6955749219134,3.40556355651458));
#19149=CARTESIAN_POINT('Ctrl Pts',(7.12670085302573,-4.11831918936923,3.48875539197247));
#19150=CARTESIAN_POINT('Ctrl Pts',(7.02192637673817,-3.49920475943206,3.57233609217612));
#19151=CARTESIAN_POINT('Ctrl Pts',(6.60200480535371,-3.02877356919622,3.65627071403784));
#19152=CARTESIAN_POINT('Ctrl Pts',(5.99389696970595,-2.85326346917548,3.74052223770667));
#19153=CARTESIAN_POINT('Ctrl Pts',(5.38356210524816,-3.02876561374954,3.82505176545516));
#19154=CARTESIAN_POINT('Ctrl Pts',(4.97486808401256,-3.48597581907603,3.90667922332894));
#19155=CARTESIAN_POINT('Ctrl Pts',(4.87764331063032,-3.96854834063101,3.97275270796177));
#19156=CARTESIAN_POINT('Ctrl Pts',(4.93363491104256,-4.28466096216571,4.01685604464165));
#19157=CARTESIAN_POINT('Ctrl Pts',(4.99817931143911,-4.45530970670709,4.04207155735716));
#19158=CARTESIAN_POINT('Ctrl Pts',(5.12597275373369,-4.69744865131441,4.07990746653167));
#19159=CARTESIAN_POINT('Ctrl Pts',(5.42875069944469,-4.99309340796393,4.13670511444809));
#19160=CARTESIAN_POINT('Ctrl Pts',(5.97231920216535,-5.14605898976926,4.21249748606625));
#19161=CARTESIAN_POINT('Ctrl Pts',(6.52320508223107,-5.02044374257342,4.28832048254892));
#19162=CARTESIAN_POINT('Ctrl Pts',(6.91110467076896,-4.67743260856581,4.35782392841035));
#19163=CARTESIAN_POINT('Ctrl Pts',(7.09644745188598,-4.25185787791867,4.42098501720712));
#19164=CARTESIAN_POINT('Ctrl Pts',(7.11227598252982,-3.83457932502243,4.47779828333078));
#19165=CARTESIAN_POINT('Ctrl Pts',(6.97422198867159,-3.44096105119827,4.53456659991209));
#19166=CARTESIAN_POINT('Ctrl Pts',(6.67241777459347,-3.08955752755044,4.59757801617794));
#19167=CARTESIAN_POINT('Ctrl Pts',(6.20242890124212,-2.8776477149725,4.66678930738527));
#19168=CARTESIAN_POINT('Ctrl Pts',(5.64251878205079,-2.91980762281901,4.74213608937642));
#19169=CARTESIAN_POINT('Ctrl Pts',(5.2704159386044,-3.1605530148329,4.80163845364204));
#19170=CARTESIAN_POINT('Ctrl Pts',(5.0774166278585,-3.41255654376288,4.84539629257686));
#19171=CARTESIAN_POINT('Ctrl Pts',(4.95479769651029,-3.65506677262475,4.88286085266752));
#19172=CARTESIAN_POINT('Ctrl Pts',(4.89096164216428,-3.99267527518354,4.9296088561907));
#19173=CARTESIAN_POINT('Ctrl Pts',(4.9676452372308,-4.39667000889553,4.98556279567646));
#19174=CARTESIAN_POINT('Ctrl Pts',(5.18583996189851,-4.74396038265063,5.04136211338706));
#19175=CARTESIAN_POINT('Ctrl Pts',(5.51489715544512,-4.98648283834255,5.09699623582978));
#19176=CARTESIAN_POINT('Ctrl Pts',(5.90877797642046,-5.0921366099034,5.15245506500268));
#19177=CARTESIAN_POINT('Ctrl Pts',(6.31208382647452,-5.04618505638536,5.20772889790527));
#19178=CARTESIAN_POINT('Ctrl Pts',(6.79039563711824,-4.79482787477752,5.28116853494519));
#19179=CARTESIAN_POINT('Ctrl Pts',(7.14364250607538,-4.18339760328549,5.37246079320281));
#19180=CARTESIAN_POINT('Ctrl Pts',(6.95465392442801,-3.3615290602033,5.48113680479085));
#19181=CARTESIAN_POINT('Ctrl Pts',(6.37954281770185,-2.97211167108618,5.57092649504958));
#19182=CARTESIAN_POINT('Ctrl Pts',(5.85508217241069,-2.95446460563552,5.64227218334414));
#19183=CARTESIAN_POINT('Ctrl Pts',(5.44460306454923,-3.0974244576334,5.70145206942602));
#19184=CARTESIAN_POINT('Ctrl Pts',(5.09938139322235,-3.43453521092238,5.76619150122483));
#19185=CARTESIAN_POINT('Ctrl Pts',(4.94592320318296,-3.93442474869926,5.83636208316637));
#19186=CARTESIAN_POINT('Ctrl Pts',(5.03197265676116,-4.35840627465708,5.89445465107149));
#19187=CARTESIAN_POINT('Ctrl Pts',(5.19219264369348,-4.60564299044654,5.93491706685731));
#19188=CARTESIAN_POINT('Ctrl Pts',(5.30719577297855,-4.72651611720447,5.95798055540973));
#19189=CARTESIAN_POINT('Ctrl Pts',(5.50053046023923,-4.88495348501329,5.99251787759586));
#19190=CARTESIAN_POINT('Ctrl Pts',(5.85832951556707,-5.02507253962729,6.04410658286047));
#19191=CARTESIAN_POINT('Ctrl Pts',(6.32126493019694,-4.96668267597821,6.10673564915363));
#19192=CARTESIAN_POINT('Ctrl Pts',(6.67328517320073,-4.74489735077078,6.1633365491453));
#19193=CARTESIAN_POINT('Ctrl Pts',(6.89435900913716,-4.44516759248262,6.21402149084589));
#19194=CARTESIAN_POINT('Ctrl Pts',(6.99016055458223,-4.08705298460299,6.26445344730346));
#19195=CARTESIAN_POINT('Ctrl Pts',(6.94870527391535,-3.72056310115263,6.31463598339954));
#19196=CARTESIAN_POINT('Ctrl Pts',(6.77696548585144,-3.39623351183634,6.36457330966794));
#19197=CARTESIAN_POINT('Ctrl Pts',(6.50006848678236,-3.15797695360399,6.41427030439494));
#19198=CARTESIAN_POINT('Ctrl Pts',(6.15689079921747,-3.03828948600061,6.46373243937456));
#19199=CARTESIAN_POINT('Ctrl Pts',(5.73494713487383,-3.05387392617641,6.52117143017342));
#19200=CARTESIAN_POINT('Ctrl Pts',(5.30575107583077,-3.29070893773119,6.58644590514151));
#19201=CARTESIAN_POINT('Ctrl Pts',(5.04125313845857,-3.77122732190886,6.6594050878354));
#19202=CARTESIAN_POINT('Ctrl Pts',(5.06714113786846,-4.2240700226978,6.71983222627245));
#19203=CARTESIAN_POINT('Ctrl Pts',(5.22896371026909,-4.53583531846688,6.76796591127916));
#19204=CARTESIAN_POINT('Ctrl Pts',(5.42916113979845,-4.74785467675554,6.80796630808184));
#19205=CARTESIAN_POINT('Ctrl Pts',(5.714367370309,-4.89850759732021,6.85183024025803));
#19206=CARTESIAN_POINT('Ctrl Pts',(6.06253639457921,-4.93755475445945,6.89952195690528));
#19207=CARTESIAN_POINT('Ctrl Pts',(6.4565847787629,-4.83233977440753,6.95498839066731));
#19208=CARTESIAN_POINT('Ctrl Pts',(6.81022730237302,-4.51633849133825,7.01814871600544));
#19209=CARTESIAN_POINT('Ctrl Pts',(6.95706828830077,-4.00489886911992,7.08893287981098));
#19210=CARTESIAN_POINT('Ctrl Pts',(6.81021224891959,-3.49584469103884,7.15948666255227));
#19211=CARTESIAN_POINT('Ctrl Pts',(6.41592301667082,-3.14352189275395,7.22985222727915));
#19212=CARTESIAN_POINT('Ctrl Pts',(5.89582428767248,-3.0555832223308,7.30007283378182));
#19213=CARTESIAN_POINT('Ctrl Pts',(5.40914881608276,-3.25711226719962,7.37019262219717));
#19214=CARTESIAN_POINT('Ctrl Pts',(5.10471600640629,-3.68647088534127,7.4402563254545));
#19215=CARTESIAN_POINT('Ctrl Pts',(5.07493689936822,-4.21187381141773,7.51030900528994));
#19216=CARTESIAN_POINT('Ctrl Pts',(5.32972438815395,-4.67276168571651,7.58039577687912));
#19217=CARTESIAN_POINT('Ctrl Pts',(5.79102554371443,-4.92784792737786,7.65056157421906));
#19218=CARTESIAN_POINT('Ctrl Pts',(6.31826031255578,-4.89837953861158,7.72085085714204));
#19219=CARTESIAN_POINT('Ctrl Pts',(6.75020660471299,-4.59231290695902,7.79130734550421));
#19220=CARTESIAN_POINT('Ctrl Pts',(6.95334524231267,-4.10180979072915,7.86197377515194));
#19221=CARTESIAN_POINT('Ctrl Pts',(6.86452811856373,-3.57660445666216,7.93289164673106));
#19222=CARTESIAN_POINT('Ctrl Pts',(6.50822949801913,-3.17741851765368,8.00410096472273));
#19223=CARTESIAN_POINT('Ctrl Pts',(5.99202912111436,-3.02846879700038,8.07564001126929));
#19224=CARTESIAN_POINT('Ctrl Pts',(5.47262775862424,-3.1772786287127,8.14754510192845));
#19225=CARTESIAN_POINT('Ctrl Pts',(5.12396773984527,-3.56713104102442,8.21717245978697));
#19226=CARTESIAN_POINT('Ctrl Pts',(5.02465088008016,-4.0589090579052,8.28449962671212));
#19227=CARTESIAN_POINT('Ctrl Pts',(5.16664179671633,-4.52183049710153,8.34949563002517));
#19228=CARTESIAN_POINT('Ctrl Pts',(5.48622133819085,-4.83366725020512,8.40942447534479));
#19229=CARTESIAN_POINT('Ctrl Pts',(5.86625745021743,-4.9665851067969,8.4641954747342));
#19230=CARTESIAN_POINT('Ctrl Pts',(6.22997586892847,-4.95324406413884,8.5137197914407));
#19231=CARTESIAN_POINT('Ctrl Pts',(6.56523678307791,-4.80705258085916,8.56348049146453));
#19232=CARTESIAN_POINT('Ctrl Pts',(6.8252178463785,-4.54733568382595,8.61348288991823));
#19233=CARTESIAN_POINT('Ctrl Pts',(6.97306928054101,-4.20890471076454,8.6637316832973));
#19234=CARTESIAN_POINT('Ctrl Pts',(6.98712341108126,-3.83802816814003,8.7142309149468));
#19235=CARTESIAN_POINT('Ctrl Pts',(6.86409431800442,-3.4858887373625,8.76498396878373));
#19236=CARTESIAN_POINT('Ctrl Pts',(6.61968641501593,-3.20161333099039,8.81599356080702));
#19237=CARTESIAN_POINT('Ctrl Pts',(6.28663539552411,-3.02539046352671,8.8672617337013));
#19238=CARTESIAN_POINT('Ctrl Pts',(5.91032079687008,-2.98281618785264,8.9187898484193));
#19239=CARTESIAN_POINT('Ctrl Pts',(5.54261902100133,-3.08115683102349,8.97057858319571));
#19240=CARTESIAN_POINT('Ctrl Pts',(5.23470149593991,-3.30818973404657,9.02262792887906));
#19241=CARTESIAN_POINT('Ctrl Pts',(5.03002953653242,-3.63360637314209,9.07493719454492));
#19242=CARTESIAN_POINT('Ctrl Pts',(4.95795339049146,-4.01324887545392,9.12750499722226));
#19243=CARTESIAN_POINT('Ctrl Pts',(5.03008733681497,-4.39465616925505,9.18032929191999));
#19244=CARTESIAN_POINT('Ctrl Pts',(5.26037098227884,-4.76198737973904,9.23930488376548));
#19245=CARTESIAN_POINT('Ctrl Pts',(5.66815402132354,-5.02611715334513,9.30453505328307));
#19246=CARTESIAN_POINT('Ctrl Pts',(6.20031175950905,-5.06610553161693,9.37613052247429));
#19247=CARTESIAN_POINT('Ctrl Pts',(6.57211483447548,-4.89867154701958,9.43089482659667));
#19248=CARTESIAN_POINT('Ctrl Pts',(6.77268428325753,-4.71398594666241,9.46854124254023));
#19249=CARTESIAN_POINT('Ctrl Pts',(6.89732261541234,-4.56210906285714,9.4956893772699));
#19250=CARTESIAN_POINT('Ctrl Pts',(7.05743952416135,-4.25373892219051,9.54330952558428));
#19251=CARTESIAN_POINT('Ctrl Pts',(7.08681427060224,-3.7413976498585,9.61164803498953));
#19252=CARTESIAN_POINT('Ctrl Pts',(6.78743967682059,-3.19877575055479,9.69412425474241));
#19253=CARTESIAN_POINT('Ctrl Pts',(6.24245837315985,-2.89706443193603,9.77704206668623));
#19254=CARTESIAN_POINT('Ctrl Pts',(5.61746900273164,-2.93185417099466,9.86037047868398));
#19255=CARTESIAN_POINT('Ctrl Pts',(5.1042042416184,-3.29518411512121,9.94407604361117));
#19256=CARTESIAN_POINT('Ctrl Pts',(4.86233946758306,-3.8785536270643,10.0281231251224));
#19257=CARTESIAN_POINT('Ctrl Pts',(4.96816269898698,-4.50332086698013,10.1124740074888));
#19258=CARTESIAN_POINT('Ctrl Pts',(5.3915816199262,-4.97752738430232,10.1970892227568));
#19259=CARTESIAN_POINT('Ctrl Pts',(6.00397807691952,-5.15417755509278,10.281927720062));
#19260=CARTESIAN_POINT('Ctrl Pts',(6.61779621608409,-4.97752665860305,10.3669471357688));
#19261=CARTESIAN_POINT('Ctrl Pts',(7.04418758947222,-4.50057596349951,10.4521040140405));
#19262=CARTESIAN_POINT('Ctrl Pts',(7.15154318711507,-3.86917823804319,10.5373541207604));
#19263=CARTESIAN_POINT('Ctrl Pts',(6.9063217242137,-3.27712490715728,10.622652644332));
#19264=CARTESIAN_POINT('Ctrl Pts',(6.38365961018741,-2.90630232377856,10.70795449752));
#19265=CARTESIAN_POINT('Ctrl Pts',(5.74407957751689,-2.87046702674317,10.7932145497474));
#19266=CARTESIAN_POINT('Ctrl Pts',(5.18413779010185,-3.18009512220889,10.8783879953558));
#19267=CARTESIAN_POINT('Ctrl Pts',(4.87504525063398,-3.73939474085648,10.9634303821887));
#19268=CARTESIAN_POINT('Ctrl Pts',(4.9113280193628,-4.37593360867611,11.0482983399598));
#19269=CARTESIAN_POINT('Ctrl Pts',(5.27937248430205,-4.89450749674953,11.1329488708158));
#19270=CARTESIAN_POINT('Ctrl Pts',(5.86527624347711,-5.13679808752952,11.2173417295453));
#19271=CARTESIAN_POINT('Ctrl Pts',(6.48799534199112,-5.03087191620999,11.3014349903219));
#19272=CARTESIAN_POINT('Ctrl Pts',(6.95693136473707,-4.61090781293032,11.3851957485584));
#19273=CARTESIAN_POINT('Ctrl Pts',(7.07219562678886,-4.21035033769926,11.4407823887657));
#19274=CARTESIAN_POINT('Ctrl Pts',(7.07222266979228,-4.00946826992833,11.4685145081909));
#19275=CARTESIAN_POINT('Origin',(7.,-4.,11.4));
#19276=CARTESIAN_POINT('Origin',(7.,-4.,11.4));
#19277=CARTESIAN_POINT('Origin',(7.,-4.,2.7));
#22312=UNCERTAINTY_MEASURE_WITH_UNIT(LENGTH_MEASURE(0.001),#22395,
'DISTANCE_ACCURACY_VALUE',
'Maximum model space distance between geometric entities at asserted c
onnectivities');
#22343=UNCERTAINTY_MEASURE_WITH_UNIT(LENGTH_MEASURE(0.001),#22395,
'DISTANCE_ACCURACY_VALUE',
'Maximum model space distance between geometric entities at asserted c
onnectivities');
#22363=(
GEOMETRIC_REPRESENTATION_CONTEXT(3)
GLOBAL_UNCERTAINTY_ASSIGNED_CONTEXT((#22312))
GLOBAL_UNIT_ASSIGNED_CONTEXT((#22395,#22397,#22398))
REPRESENTATION_CONTEXT('','3D')
);
#22394=(
GEOMETRIC_REPRESENTATION_CONTEXT(3)
GLOBAL_UNCERTAINTY_ASSIGNED_CONTEXT((#22343))
GLOBAL_UNIT_ASSIGNED_CONTEXT((#22395,#22397,#22398))
REPRESENTATION_CONTEXT('','3D')
);
#22395=(
LENGTH_UNIT()
NAMED_UNIT(*)
SI_UNIT(.CENTI.,.METRE.)
);
#22397=(
NAMED_UNIT(*)
PLANE_ANGLE_UNIT()
SI_UNIT($,.RADIAN.)
);
#22398=(
NAMED_UNIT(*)
SI_UNIT($,.STERADIAN.)
SOLID_ANGLE_UNIT()
);
#22418=SHAPE_DEFINITION_REPRESENTATION(#22468,#22657);
#22468=PRODUCT_DEFINITION_SHAPE('',$,#22708);
#22657=SHAPE_REPRESENTATION('',(#10137),#22363);
#22688=PRODUCT_DEFINITION_CONTEXT('part definition',#22840,'design');
#22708=PRODUCT_DEFINITION('Installed compression spring (2)',
'Installed compression spring (2)',#22758,#22688);
#22758=PRODUCT_DEFINITION_FORMATION('',$,#22861);
#22840=APPLICATION_CONTEXT(
'Core Data for Automotive Mechanical Design Process');
#22841=PRODUCT_CONTEXT('part definition',#22840,'mechanical');
#22861=PRODUCT('Installed compression spring (2)',
'Installed compression spring (2)','Installed compression spring (2)',(#22841));
#22955=COLOUR_RGB('Grey',0.48,0.52,0.57);
#22956=FILL_AREA_STYLE_COLOUR('',#22955);
#22957=FILL_AREA_STYLE('',(#22956));
#22958=SURFACE_STYLE_FILL_AREA(#22957);
#22959=SURFACE_SIDE_STYLE('',(#22958));
#22960=SURFACE_STYLE_USAGE(.BOTH.,#22959);
#22961=PRESENTATION_STYLE_ASSIGNMENT((#22960));
ENDSEC;
END-ISO-10303-21;
